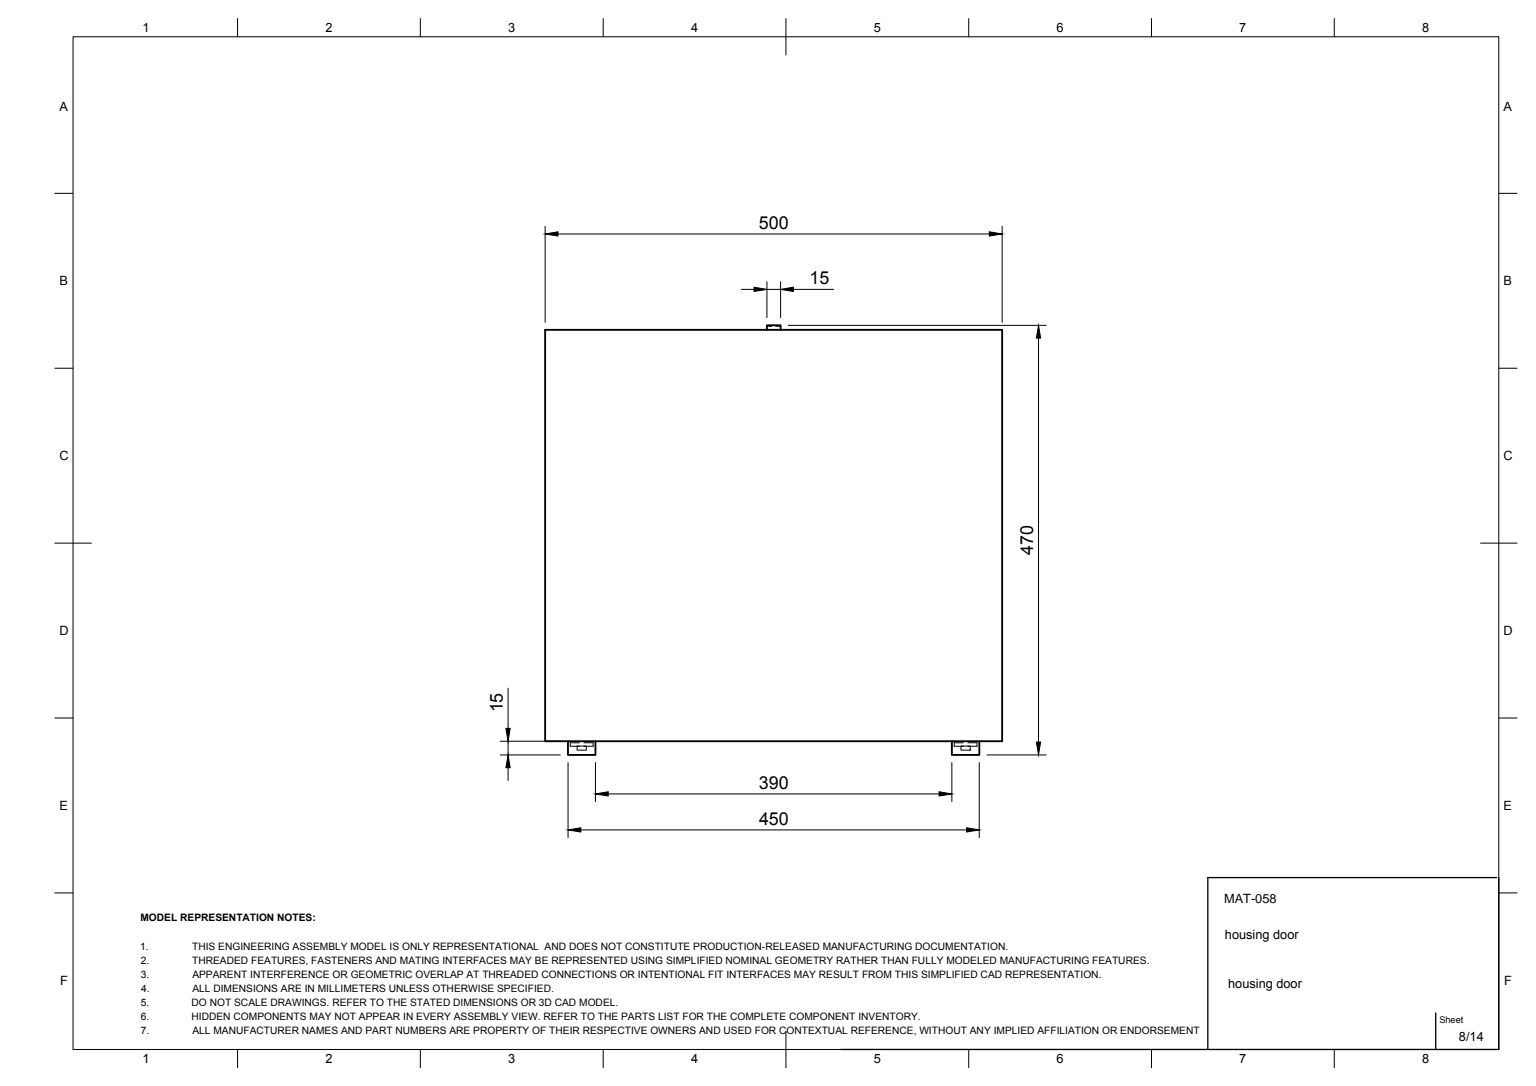
ISO-10303-21;
HEADER;
FILE_DESCRIPTION (('STEP AP214'),
    '1' );
FILE_NAME ('housing door.step',
    '2026-10-21T17:54:40',
    ( '' ),
    ( '' ),
    'SwSTEP 2.0',
    'SolidWorks 2026',
    '' );
FILE_SCHEMA (( 'AUTOMOTIVE_DESIGN' ));
ENDSEC;

DATA;
#107=VECTOR ( 'NONE', #36359, 1000.000000000000000 ) ;
#131=DIRECTION ( 'NONE',  ( -1.000000000000000000, -1.156482317317870492E-16, 0.000000000000000000 ) ) ;
#169=VERTEX_POINT ( 'NONE', #24652 ) ;
#257=LINE ( 'NONE', #31044, #20090 ) ;
#265=LINE ( 'NONE', #19995, #41034 ) ;
#282=DIRECTION ( 'NONE',  ( 0.000000000000000000, -0.000000000000000000, 1.000000000000000000 ) ) ;
#297=VERTEX_POINT ( 'NONE', #25154 ) ;
#306=EDGE_CURVE ( 'NONE', #36749, #10540, #17931, .T. ) ;
#342=ADVANCED_FACE ( 'NONE', ( #29249, #10502, #26150 ), #6152, .F. ) ;
#434=VECTOR ( 'NONE', #13236, 1000.000000000000000 ) ;
#444=FACE_OUTER_BOUND ( 'NONE', #40389, .T. ) ;
#536=EDGE_CURVE ( 'NONE', #38434, #12843, #25274, .T. ) ;
#613=PRODUCT_DEFINITION_CONTEXT ( 'detailed design', #38126, 'design' ) ;
#675=DIRECTION ( 'NONE',  ( 1.000000000000000000, -0.000000000000000000, -0.000000000000000000 ) ) ;
#692=VERTEX_POINT ( 'NONE', #29376 ) ;
#720=LINE ( 'NONE', #35138, #11092 ) ;
#772=DIRECTION ( 'NONE',  ( 0.000000000000000000, 1.000000000000000000, 0.000000000000000000 ) ) ;
#838=DIRECTION ( 'NONE',  ( -1.156482317317870492E-16, 1.000000000000000000, 0.000000000000000000 ) ) ;
#856=ORIENTED_EDGE ( 'NONE', *, *, #7061, .T. ) ;
#953=VERTEX_POINT ( 'NONE', #13403 ) ;
#966=ORIENTED_EDGE ( 'NONE', *, *, #43724, .T. ) ;
#983=VECTOR ( 'NONE', #33572, 1000.000000000000000 ) ;
#1078=( GEOMETRIC_REPRESENTATION_CONTEXT ( 3 ) GLOBAL_UNCERTAINTY_ASSIGNED_CONTEXT ( ( #42989 ) ) GLOBAL_UNIT_ASSIGNED_CONTEXT ( ( #15335, #42505, #10210 ) ) REPRESENTATION_CONTEXT ( 'NONE', 'WORKASPACE' ) );
#1106=FACE_OUTER_BOUND ( 'NONE', #15806, .T. ) ;
#1128=FACE_OUTER_BOUND ( 'NONE', #22979, .T. ) ;
#1143=CARTESIAN_POINT ( 'NONE',  ( 10.00000000000000000, -250.0000000000000000, 225.0000000000000000 ) ) ;
#1154=VECTOR ( 'NONE', #48411, 1000.000000000000000 ) ;
#1155=CARTESIAN_POINT ( 'NONE',  ( 2.499999999999956035, -194.9999999999999716, -224.9999999999999716 ) ) ;
#1205=PLANE ( 'NONE',  #27858 ) ;
#1231=EDGE_CURVE ( 'NONE', #28520, #3732, #42617, .T. ) ;
#1249=DIRECTION ( 'NONE',  ( -0.000000000000000000, -0.000000000000000000, 1.000000000000000000 ) ) ;
#1261=CARTESIAN_POINT ( 'NONE',  ( -8.760073316077686911, -197.4999999999999432, -228.6347188485896140 ) ) ;
#1360=VECTOR ( 'NONE', #42599, 1000.000000000000000 ) ;
#1476=LINE ( 'NONE', #17109, #47212 ) ;
#1506=DIRECTION ( 'NONE',  ( 0.000000000000000000, 0.000000000000000000, 1.000000000000000000 ) ) ;
#1525=ORIENTED_EDGE ( 'NONE', *, *, #2062, .T. ) ;
#1538=LINE ( 'NONE', #40533, #35833 ) ;
#1568=DIRECTION ( 'NONE',  ( 1.000000000000000000, 8.673617379884028076E-17, -0.000000000000000000 ) ) ;
#1577=CARTESIAN_POINT ( 'NONE',  ( 6.204997580903516941, 7.611558401714507482, 225.0000000000000000 ) ) ;
#1621=PLANE ( 'NONE',  #37359 ) ;
#1642=CARTESIAN_POINT ( 'NONE',  ( 2.500000000000000444, 224.9999999999999716, -240.0000000000000000 ) ) ;
#1750=ADVANCED_FACE ( 'NONE', ( #36154 ), #24355, .T. ) ;
#1761=ORIENTED_EDGE ( 'NONE', *, *, #13263, .F. ) ;
#1812=AXIS2_PLACEMENT_3D ( 'NONE', #17777, #25735, #6236 ) ;
#1820=DIRECTION ( 'NONE',  ( 1.000000000000000000, -0.000000000000000000, -0.000000000000000000 ) ) ;
#1892=EDGE_CURVE ( 'NONE', #41332, #44274, #10449, .T. ) ;
#1916=VECTOR ( 'NONE', #48903, 1000.000000000000000 ) ;
#1923=DIRECTION ( 'NONE',  ( 0.000000000000000000, 1.000000000000000000, 0.000000000000000000 ) ) ;
#2017=DIRECTION ( 'NONE',  ( 0.000000000000000000, -1.000000000000000000, 0.000000000000000000 ) ) ;
#2029=DIRECTION ( 'NONE',  ( -1.000000000000000000, 0.000000000000000000, -0.000000000000000000 ) ) ;
#2049=CARTESIAN_POINT ( 'NONE',  ( 7.500000000000000000, 224.9999999999999716, -240.0000000000000000 ) ) ;
#2057=AXIS2_PLACEMENT_3D ( 'NONE', #20662, #32722, #16822 ) ;
#2062=EDGE_CURVE ( 'NONE', #44581, #5075, #47588, .T. ) ;
#2090=FACE_OUTER_BOUND ( 'NONE', #16667, .T. ) ;
#2124=ORIENTED_EDGE ( 'NONE', *, *, #7316, .T. ) ;
#2180=EDGE_CURVE ( 'NONE', #169, #35061, #50319, .T. ) ;
#2216=ORIENTED_EDGE ( 'NONE', *, *, #21301, .F. ) ;
#2233=ORIENTED_EDGE ( 'NONE', *, *, #16780, .F. ) ;
#2234=ADVANCED_FACE ( 'NONE', ( #38594 ), #34751, .T. ) ;
#2362=CARTESIAN_POINT ( 'NONE',  ( -4.999999999999948486, -204.9999999999999716, -234.7500000000000000 ) ) ;
#2397=EDGE_LOOP ( 'NONE', ( #43510, #31402, #50616, #4938 ) ) ;
#2414=VERTEX_POINT ( 'NONE', #19238 ) ;
#2509=LINE ( 'NONE', #25356, #48276 ) ;
#2601=VERTEX_POINT ( 'NONE', #27716 ) ;
#2611=CARTESIAN_POINT ( 'NONE',  ( 4.204997580903516941, -7.388441598285492518, 229.0000000000000000 ) ) ;
#2649=DIRECTION ( 'NONE',  ( 0.000000000000000000, -0.000000000000000000, 1.000000000000000000 ) ) ;
#2666=EDGE_LOOP ( 'NONE', ( #26311, #43649, #8617, #21048 ) ) ;
#2736=PLANE ( 'NONE',  #28390 ) ;
#2783=ORIENTED_EDGE ( 'NONE', *, *, #20337, .F. ) ;
#2843=LINE ( 'NONE', #46433, #10000 ) ;
#2855=VECTOR ( 'NONE', #2017, 1000.000000000000000 ) ;
#2865=VECTOR ( 'NONE', #35878, 1000.000000000000000 ) ;
#2880=VERTEX_POINT ( 'NONE', #11947 ) ;
#3028=CARTESIAN_POINT ( 'NONE',  ( -22.82242230425432439, -2.816136035261162185, 226.0000000000000000 ) ) ;
#3077=ORIENTED_EDGE ( 'NONE', *, *, #19358, .F. ) ;
#3156=VERTEX_POINT ( 'NONE', #34744 ) ;
#3185=LINE ( 'NONE', #27833, #40241 ) ;
#3357=ORIENTED_EDGE ( 'NONE', *, *, #36236, .F. ) ;
#3367=LINE ( 'NONE', #34699, #44682 ) ;
#3415=CARTESIAN_POINT ( 'NONE',  ( -22.82242230425432439, -2.816136035261162185, 229.0000000000000000 ) ) ;
#3446=VERTEX_POINT ( 'NONE', #28795 ) ;
#3504=CARTESIAN_POINT ( 'NONE',  ( 2.500000000000000444, 224.9999999999999716, -240.0000000000000000 ) ) ;
#3509=DIRECTION ( 'NONE',  ( -1.156482317317870492E-16, 1.000000000000000000, 0.000000000000000000 ) ) ;
#3532=EDGE_LOOP ( 'NONE', ( #13431, #22172, #30047, #39452 ) ) ;
#3567=EDGE_CURVE ( 'NONE', #3732, #45897, #46674, .T. ) ;
#3641=AXIS2_PLACEMENT_3D ( 'NONE', #40376, #16766, #8571 ) ;
#3642=CARTESIAN_POINT ( 'NONE',  ( -4.999999999999997335, 204.9999999999999716, -234.7500000000000000 ) ) ;
#3659=ORIENTED_EDGE ( 'NONE', *, *, #49978, .F. ) ;
#3690=CARTESIAN_POINT ( 'NONE',  ( 2.500000000000001776, 214.9999999999999716, -234.7500000000000000 ) ) ;
#3732=VERTEX_POINT ( 'NONE', #47181 ) ;
#3750=LINE ( 'NONE', #31734, #13278 ) ;
#3784=DIRECTION ( 'NONE',  ( -1.000000000000000000, 0.000000000000000000, 0.000000000000000000 ) ) ;
#3839=DIRECTION ( 'NONE',  ( -1.156482317317870492E-16, 1.000000000000000000, 0.000000000000000000 ) ) ;
#3858=DIRECTION ( 'NONE',  ( -0.000000000000000000, 1.000000000000000000, 0.000000000000000000 ) ) ;
#3871=PLANE ( 'NONE',  #11659 ) ;
#3881=PLANE ( 'NONE',  #7841 ) ;
#3891=EDGE_CURVE ( 'NONE', #27411, #18811, #40534, .T. ) ;
#3986=EDGE_CURVE ( 'NONE', #17007, #4976, #15098, .T. ) ;
#4136=CARTESIAN_POINT ( 'NONE',  ( 4.204997580903516941, -7.388441598285492518, 229.0000000000000000 ) ) ;
#4192=EDGE_CURVE ( 'NONE', #26282, #2880, #7924, .T. ) ;
#4231=VECTOR ( 'NONE', #24839, 1000.000000000000000 ) ;
#4341=EDGE_CURVE ( 'NONE', #22510, #5553, #36863, .T. ) ;
#4359=CARTESIAN_POINT ( 'NONE',  ( 4.204997580903515164, -7.388441598285492518, 229.0000000000000000 ) ) ;
#4372=FACE_OUTER_BOUND ( 'NONE', #5239, .T. ) ;
#4545=ORIENTED_EDGE ( 'NONE', *, *, #25529, .T. ) ;
#4570=DIRECTION ( 'NONE',  ( -1.445602896647339410E-16, -1.000000000000000000, -0.000000000000000000 ) ) ;
#4620=ORIENTED_EDGE ( 'NONE', *, *, #5814, .T. ) ;
#4643=FACE_OUTER_BOUND ( 'NONE', #22886, .T. ) ;
#4647=VECTOR ( 'NONE', #1923, 1000.000000000000000 ) ;
#4742=LINE ( 'NONE', #47550, #10008 ) ;
#4752=EDGE_LOOP ( 'NONE', ( #20974, #12743, #21409, #26520 ) ) ;
#4768=LINE ( 'NONE', #15816, #17470 ) ;
#4857=ORIENTED_EDGE ( 'NONE', *, *, #10866, .F. ) ;
#4894=DIRECTION ( 'NONE',  ( 0.000000000000000000, 0.000000000000000000, -1.000000000000000000 ) ) ;
#4938=ORIENTED_EDGE ( 'NONE', *, *, #6764, .F. ) ;
#4976=VERTEX_POINT ( 'NONE', #2049 ) ;
#4998=VECTOR ( 'NONE', #29646, 1000.000000000000000 ) ;
#5035=EDGE_LOOP ( 'NONE', ( #12053, #2783, #27028, #33906 ) ) ;
#5052=VERTEX_POINT ( 'NONE', #42794 ) ;
#5075=VERTEX_POINT ( 'NONE', #31025 ) ;
#5193=DIRECTION ( 'NONE',  ( -1.000000000000000000, 0.000000000000000000, 0.000000000000000000 ) ) ;
#5206=LINE ( 'NONE', #20851, #28066 ) ;
#5239=EDGE_LOOP ( 'NONE', ( #45106, #33408, #44020, #33929 ) ) ;
#5289=APPLICATION_CONTEXT ( 'automotive_design' ) ;
#5291=VERTEX_POINT ( 'NONE', #41228 ) ;
#5307=VERTEX_POINT ( 'NONE', #13016 ) ;
#5329=LINE ( 'NONE', #29437, #38449 ) ;
#5330=LINE ( 'NONE', #20729, #45365 ) ;
#5331=AXIS2_PLACEMENT_3D ( 'NONE', #44627, #1568, #5655 ) ;
#5338=CIRCLE ( 'NONE', #38104, 1.880036658038868103 ) ;
#5379=CARTESIAN_POINT ( 'NONE',  ( -8.760073316077734873, 222.4999999999999716, -228.6347188485896140 ) ) ;
#5407=ORIENTED_EDGE ( 'NONE', *, *, #2180, .F. ) ;
#5435=FACE_OUTER_BOUND ( 'NONE', #31932, .T. ) ;
#5466=CARTESIAN_POINT ( 'NONE',  ( 4.204997580903516941, 7.611558401714507482, 229.0000000000000000 ) ) ;
#5471=CARTESIAN_POINT ( 'NONE',  ( -4.999999999999948486, -204.9999999999999716, -234.7500000000000000 ) ) ;
#5481=EDGE_CURVE ( 'NONE', #10540, #15922, #15557, .T. ) ;
#5492=VECTOR ( 'NONE', #44100, 1000.000000000000000 ) ;
#5506=PLANE ( 'NONE',  #6884 ) ;
#5507=EDGE_CURVE ( 'NONE', #2601, #43558, #3750, .T. ) ;
#5553=VERTEX_POINT ( 'NONE', #20920 ) ;
#5559=EDGE_CURVE ( 'NONE', #15591, #13831, #33489, .T. ) ;
#5616=DIRECTION ( 'NONE',  ( 1.000000000000000000, 0.000000000000000000, -0.000000000000000000 ) ) ;
#5655=DIRECTION ( 'NONE',  ( -8.673617379884028076E-17, 1.000000000000000000, 0.000000000000000000 ) ) ;
#5737=ORIENTED_EDGE ( 'NONE', *, *, #39075, .F. ) ;
#5814=EDGE_CURVE ( 'NONE', #3446, #692, #48217, .T. ) ;
#5862=CARTESIAN_POINT ( 'NONE',  ( 10.00000000000000000, -250.0000000000000000, 225.0000000000000000 ) ) ;
#5922=DIRECTION ( 'NONE',  ( 1.000000000000000000, 0.000000000000000000, 0.000000000000000000 ) ) ;
#5952=DIRECTION ( 'NONE',  ( 1.000000000000000000, 0.000000000000000000, -0.000000000000000000 ) ) ;
#6047=CARTESIAN_POINT ( 'NONE',  ( 7.499999999999944045, -224.9999999999999716, -240.0000000000000000 ) ) ;
#6093=DIRECTION ( 'NONE',  ( -1.000000000000000000, -0.000000000000000000, -0.000000000000000000 ) ) ;
#6112=ORIENTED_EDGE ( 'NONE', *, *, #7061, .F. ) ;
#6152=PLANE ( 'NONE',  #17129 ) ;
#6236=DIRECTION ( 'NONE',  ( 1.000000000000000000, 0.000000000000000000, 0.000000000000000000 ) ) ;
#6260=ORIENTED_EDGE ( 'NONE', *, *, #48354, .T. ) ;
#6264=EDGE_CURVE ( 'NONE', #4976, #14400, #22504, .T. ) ;
#6528=DIRECTION ( 'NONE',  ( 0.000000000000000000, 1.000000000000000000, 0.000000000000000000 ) ) ;
#6543=AXIS2_PLACEMENT_3D ( 'NONE', #40334, #838, #35755 ) ;
#6560=DIRECTION ( 'NONE',  ( 1.000000000000000000, 1.156482317317870492E-16, -0.000000000000000000 ) ) ;
#6576=VECTOR ( 'NONE', #772, 1000.000000000000000 ) ;
#6634=LINE ( 'NONE', #3028, #34072 ) ;
#6647=CARTESIAN_POINT ( 'NONE',  ( 0.000000000000000000, -250.0000000000000000, 225.0000000000000000 ) ) ;
#6649=DIRECTION ( 'NONE',  ( 0.000000000000000000, 0.000000000000000000, 1.000000000000000000 ) ) ;
#6660=AXIS2_PLACEMENT_3D ( 'NONE', #29673, #25323, #45293 ) ;
#6677=EDGE_CURVE ( 'NONE', #29935, #41724, #47839, .T. ) ;
#6764=EDGE_CURVE ( 'NONE', #13831, #12618, #18088, .T. ) ;
#6798=EDGE_CURVE ( 'NONE', #38906, #36749, #3185, .T. ) ;
#6824=EDGE_CURVE ( 'NONE', #47608, #35061, #42694, .T. ) ;
#6867=LINE ( 'NONE', #41011, #31966 ) ;
#6878=ADVANCED_FACE ( 'NONE', ( #30668 ), #15010, .T. ) ;
#6884=AXIS2_PLACEMENT_3D ( 'NONE', #29867, #21403, #32979 ) ;
#6886=DIRECTION ( 'NONE',  ( 0.000000000000000000, 0.000000000000000000, -1.000000000000000000 ) ) ;
#6892=DIRECTION ( 'NONE',  ( -1.000000000000000000, -1.156482317317870492E-16, 0.000000000000000000 ) ) ;
#6971=EDGE_CURVE ( 'NONE', #5052, #12618, #48285, .T. ) ;
#6973=SHAPE_REPRESENTATION_RELATIONSHIP ( 'NONE' , 'NONE' ,  #41838, #12371 ) ;
#6982=ORIENTED_EDGE ( 'NONE', *, *, #1231, .F. ) ;
#7061=EDGE_CURVE ( 'NONE', #16247, #22924, #31945, .T. ) ;
#7147=CARTESIAN_POINT ( 'NONE',  ( -6.880036658038815922, -222.4999999999999716, -228.6347188485896140 ) ) ;
#7156=CARTESIAN_POINT ( 'NONE',  ( 2.499999999999948930, -214.9999999999999716, -230.2499999999999716 ) ) ;
#7175=LINE ( 'NONE', #34141, #29751 ) ;
#7204=ORIENTED_EDGE ( 'NONE', *, *, #50260, .F. ) ;
#7249=CARTESIAN_POINT ( 'NONE',  ( 21.23829395927641883, -7.388441598285492518, 230.0000000000000000 ) ) ;
#7272=CLOSED_SHELL ( 'NONE', ( #18927, #43714, #46822, #342, #22177, #23686, #28004, #1750, #42808, #41362, #48697, #26015, #11744, #28368, #23224, #43415, #21259, #19388, #38381, #50269, #18972, #16515, #14568, #10938, #44795, #41279, #17789, #42653, #44036, #37273, #10881, #10910, #41826, #39115, #8876, #16811, #36818 ) ) ;
#7316=EDGE_CURVE ( 'NONE', #21384, #9147, #38320, .T. ) ;
#7436=CARTESIAN_POINT ( 'NONE',  ( 10.00000000000000000, 249.9999999999999716, -224.9999999999999716 ) ) ;
#7496=DIRECTION ( 'NONE',  ( -1.000000000000000000, 0.000000000000000000, 0.000000000000000000 ) ) ;
#7504=PLANE ( 'NONE',  #45239 ) ;
#7549=ORIENTED_EDGE ( 'NONE', *, *, #2180, .T. ) ;
#7556=ORIENTED_EDGE ( 'NONE', *, *, #13570, .F. ) ;
#7588=VECTOR ( 'NONE', #27240, 1000.000000000000000 ) ;
#7601=EDGE_CURVE ( 'NONE', #17007, #3446, #30468, .T. ) ;
#7614=DIRECTION ( 'NONE',  ( -0.000000000000000000, -1.000000000000000000, -0.000000000000000000 ) ) ;
#7697=EDGE_CURVE ( 'NONE', #44581, #45897, #24309, .T. ) ;
#7779=CARTESIAN_POINT ( 'NONE',  ( 2.499999999999945377, -224.9999999999999716, -240.0000000000000000 ) ) ;
#7813=DIRECTION ( 'NONE',  ( 0.000000000000000000, 0.000000000000000000, 1.000000000000000000 ) ) ;
#7841=AXIS2_PLACEMENT_3D ( 'NONE', #31092, #11332, #39302 ) ;
#7895=DIRECTION ( 'NONE',  ( 1.000000000000000000, -0.000000000000000000, 0.000000000000000000 ) ) ;
#7924=LINE ( 'NONE', #43040, #21221 ) ;
#7957=ORIENTED_EDGE ( 'NONE', *, *, #5507, .T. ) ;
#7958=DIRECTION ( 'NONE',  ( -1.000000000000000000, 0.000000000000000000, 0.000000000000000000 ) ) ;
#8031=LINE ( 'NONE', #7779, #37794 ) ;
#8047=DIRECTION ( 'NONE',  ( 1.156482317317870492E-16, -1.000000000000000000, -0.000000000000000000 ) ) ;
#8219=ORIENTED_EDGE ( 'NONE', *, *, #22109, .F. ) ;
#8269=VECTOR ( 'NONE', #50154, 1000.000000000000000 ) ;
#8273=EDGE_CURVE ( 'NONE', #42084, #26449, #22648, .T. ) ;
#8306=ORIENTED_EDGE ( 'NONE', *, *, #6971, .T. ) ;
#8451=DIRECTION ( 'NONE',  ( -1.156482317317871478E-16, 1.000000000000000000, -0.000000000000000000 ) ) ;
#8503=ORIENTED_EDGE ( 'NONE', *, *, #31244, .T. ) ;
#8538=ORIENTED_EDGE ( 'NONE', *, *, #37613, .F. ) ;
#8571=DIRECTION ( 'NONE',  ( 1.000000000000000000, 0.000000000000000000, -0.000000000000000000 ) ) ;
#8586=EDGE_CURVE ( 'NONE', #26976, #25838, #9043, .T. ) ;
#8613=ORIENTED_EDGE ( 'NONE', *, *, #16112, .F. ) ;
#8615=CARTESIAN_POINT ( 'NONE',  ( -4.999999999999948486, -214.9999999999999716, -230.2499999999999716 ) ) ;
#8617=ORIENTED_EDGE ( 'NONE', *, *, #4192, .T. ) ;
#8681=AXIS2_PLACEMENT_3D ( 'NONE', #28105, #43741, #16556 ) ;
#8685=VECTOR ( 'NONE', #31298, 1000.000000000000000 ) ;
#8714=ORIENTED_EDGE ( 'NONE', *, *, #9844, .T. ) ;
#8715=AXIS2_PLACEMENT_3D ( 'NONE', #21023, #21270, #13060 ) ;
#8773=FACE_BOUND ( 'NONE', #2397, .T. ) ;
#8832=ORIENTED_EDGE ( 'NONE', *, *, #9531, .T. ) ;
#8834=DIRECTION ( 'NONE',  ( -0.000000000000000000, -0.000000000000000000, -1.000000000000000000 ) ) ;
#8845=VECTOR ( 'NONE', #6093, 1000.000000000000000 ) ;
#8876=ADVANCED_FACE ( 'NONE', ( #20512 ), #48421, .F. ) ;
#8899=EDGE_CURVE ( 'NONE', #36068, #2414, #44097, .T. ) ;
#8927=LINE ( 'NONE', #32295, #21492 ) ;
#8946=FACE_OUTER_BOUND ( 'NONE', #24191, .T. ) ;
#8950=ORIENTED_EDGE ( 'NONE', *, *, #32185, .F. ) ;
#8961=ORIENTED_EDGE ( 'NONE', *, *, #7697, .F. ) ;
#9043=CIRCLE ( 'NONE', #6543, 1.880036658038868991 ) ;
#9058=EDGE_LOOP ( 'NONE', ( #13653, #11756, #9966, #7204 ) ) ;
#9069=AXIS2_PLACEMENT_3D ( 'NONE', #47158, #3839, #7958 ) ;
#9147=VERTEX_POINT ( 'NONE', #42027 ) ;
#9158=ORIENTED_EDGE ( 'NONE', *, *, #306, .F. ) ;
#9318=PLANE ( 'NONE',  #11909 ) ;
#9353=CARTESIAN_POINT ( 'NONE',  ( -4.999999999999948486, -204.9999999999999716, -234.7500000000000000 ) ) ;
#9358=ORIENTED_EDGE ( 'NONE', *, *, #6264, .T. ) ;
#9445=( GEOMETRIC_REPRESENTATION_CONTEXT ( 3 ) GLOBAL_UNCERTAINTY_ASSIGNED_CONTEXT ( ( #27008 ) ) GLOBAL_UNIT_ASSIGNED_CONTEXT ( ( #18758, #33681, #45182 ) ) REPRESENTATION_CONTEXT ( 'NONE', 'WORKASPACE' ) );
#9531=EDGE_CURVE ( 'NONE', #26103, #43683, #44893, .T. ) ;
#9576=FACE_OUTER_BOUND ( 'NONE', #11976, .T. ) ;
#9607=ORIENTED_EDGE ( 'NONE', *, *, #45706, .T. ) ;
#9743=AXIS2_PLACEMENT_3D ( 'NONE', #22243, #21987, #37661 ) ;
#9779=DIRECTION ( 'NONE',  ( -1.156482317317870492E-16, 1.000000000000000000, 0.000000000000000000 ) ) ;
#9795=CARTESIAN_POINT ( 'NONE',  ( -4.999999999999948486, -204.9999999999999716, -234.7500000000000000 ) ) ;
#9844=EDGE_CURVE ( 'NONE', #29454, #17433, #49610, .T. ) ;
#9893=EDGE_LOOP ( 'NONE', ( #38931, #16511, #24800, #25278 ) ) ;
#9966=ORIENTED_EDGE ( 'NONE', *, *, #10574, .F. ) ;
#10000=VECTOR ( 'NONE', #50518, 1000.000000000000000 ) ;
#10008=VECTOR ( 'NONE', #16046, 1000.000000000000000 ) ;
#10164=ORIENTED_EDGE ( 'NONE', *, *, #19288, .T. ) ;
#10210=( NAMED_UNIT ( * ) SI_UNIT ( $, .STERADIAN. ) SOLID_ANGLE_UNIT ( ) );
#10235=DIRECTION ( 'NONE',  ( -0.000000000000000000, -0.000000000000000000, 1.000000000000000000 ) ) ;
#10269=ORIENTED_EDGE ( 'NONE', *, *, #50260, .T. ) ;
#10275=LINE ( 'NONE', #48717, #16601 ) ;
#10308=CARTESIAN_POINT ( 'NONE',  ( 7.500000000000000000, 224.9999999999999716, -240.0000000000000000 ) ) ;
#10339=CARTESIAN_POINT ( 'NONE',  ( 7.499999999999944045, -224.9999999999999716, -240.0000000000000000 ) ) ;
#10449=LINE ( 'NONE', #48891, #24716 ) ;
#10485=EDGE_LOOP ( 'NONE', ( #27195, #11760, #38471, #31246 ) ) ;
#10502=FACE_OUTER_BOUND ( 'NONE', #3532, .T. ) ;
#10540=VERTEX_POINT ( 'NONE', #29291 ) ;
#10559=CARTESIAN_POINT ( 'NONE',  ( -4.999999999999948486, -204.9999999999999716, -230.2499999999999716 ) ) ;
#10574=EDGE_CURVE ( 'NONE', #17433, #3732, #43919, .T. ) ;
#10608=ORIENTED_EDGE ( 'NONE', *, *, #33976, .T. ) ;
#10623=PLANE ( 'NONE',  #40550 ) ;
#10677=CARTESIAN_POINT ( 'NONE',  ( -6.880036658038864772, 197.4999999999999432, -228.6347188485896140 ) ) ;
#10807=LINE ( 'NONE', #23115, #32955 ) ;
#10866=EDGE_CURVE ( 'NONE', #15922, #26103, #25136, .T. ) ;
#10871=CARTESIAN_POINT ( 'NONE',  ( 6.204997580903516941, -7.388441598285492518, 230.0000000000000000 ) ) ;
#10881=ADVANCED_FACE ( 'NONE', ( #20764, #13062 ), #28729, .T. ) ;
#10910=ADVANCED_FACE ( 'NONE', ( #24877, #32334 ), #40528, .T. ) ;
#10921=LINE ( 'NONE', #38396, #11054 ) ;
#10938=ADVANCED_FACE ( 'NONE', ( #26124 ), #45605, .F. ) ;
#11054=VECTOR ( 'NONE', #25827, 1000.000000000000000 ) ;
#11071=EDGE_LOOP ( 'NONE', ( #13031, #28160, #2124, #24857, #5737, #16254 ) ) ;
#11092=VECTOR ( 'NONE', #11511, 1000.000000000000000 ) ;
#11217=EDGE_CURVE ( 'NONE', #19049, #22510, #1476, .T. ) ;
#11242=ORIENTED_EDGE ( 'NONE', *, *, #26808, .T. ) ;
#11312=DIRECTION ( 'NONE',  ( 0.000000000000000000, 0.000000000000000000, 1.000000000000000000 ) ) ;
#11332=DIRECTION ( 'NONE',  ( -1.000000000000000000, 0.000000000000000000, 0.000000000000000000 ) ) ;
#11358=ORIENTED_EDGE ( 'NONE', *, *, #39075, .T. ) ;
#11511=DIRECTION ( 'NONE',  ( -1.000000000000000000, -0.000000000000000000, -0.000000000000000000 ) ) ;
#11514=LINE ( 'NONE', #39487, #20879 ) ;
#11659=AXIS2_PLACEMENT_3D ( 'NONE', #4136, #19509, #27234 ) ;
#11664=AXIS2_PLACEMENT_3D ( 'NONE', #20012, #3858, #282 ) ;
#11690=ORIENTED_EDGE ( 'NONE', *, *, #19101, .F. ) ;
#11727=PLANE ( 'NONE',  #34672 ) ;
#11744=ADVANCED_FACE ( 'NONE', ( #5435 ), #21339, .F. ) ;
#11746=ORIENTED_EDGE ( 'NONE', *, *, #7316, .F. ) ;
#11756=ORIENTED_EDGE ( 'NONE', *, *, #3567, .F. ) ;
#11760=ORIENTED_EDGE ( 'NONE', *, *, #7601, .F. ) ;
#11797=AXIS2_PLACEMENT_3D ( 'NONE', #44343, #45092, #44840 ) ;
#11893=CARTESIAN_POINT ( 'NONE',  ( 2.499999999999945377, -224.9999999999999716, -240.0000000000000000 ) ) ;
#11909=AXIS2_PLACEMENT_3D ( 'NONE', #16765, #32424, #48018 ) ;
#11947=CARTESIAN_POINT ( 'NONE',  ( -22.82242230425432439, -2.816136035261162185, 230.0000000000000000 ) ) ;
#11968=DIRECTION ( 'NONE',  ( -1.000000000000000000, 0.000000000000000000, 0.000000000000000000 ) ) ;
#11976=EDGE_LOOP ( 'NONE', ( #8832, #50636, #31082, #21291 ) ) ;
#11980=CARTESIAN_POINT ( 'NONE',  ( -4.999999999999997335, 204.9999999999999716, -230.2499999999999716 ) ) ;
#12053=ORIENTED_EDGE ( 'NONE', *, *, #19288, .F. ) ;
#12117=ORIENTED_EDGE ( 'NONE', *, *, #38802, .F. ) ;
#12139=ORIENTED_EDGE ( 'NONE', *, *, #22804, .T. ) ;
#12230=CARTESIAN_POINT ( 'NONE',  ( -7.822422304254325276, -2.816136035261162185, 226.0000000000000000 ) ) ;
#12339=LINE ( 'NONE', #12851, #30480 ) ;
#12371=ADVANCED_BREP_SHAPE_REPRESENTATION ( '', ( #38799, #38969, #38632, #45486 ), #9445 ) ;
#12389=ORIENTED_EDGE ( 'NONE', *, *, #16780, .T. ) ;
#12390=VECTOR ( 'NONE', #36354, 1000.000000000000000 ) ;
#12409=ORIENTED_EDGE ( 'NONE', *, *, #11217, .F. ) ;
#12420=AXIS2_PLACEMENT_3D ( 'NONE', #10339, #33196, #18259 ) ;
#12439=ORIENTED_EDGE ( 'NONE', *, *, #10574, .T. ) ;
#12443=CYLINDRICAL_SURFACE ( 'NONE', #8681, 1.880036658038868103 ) ;
#12456=PLANE ( 'NONE',  #2057 ) ;
#12487=CARTESIAN_POINT ( 'NONE',  ( 6.204997580903516941, 7.611558401714507482, 230.0000000000000000 ) ) ;
#12498=CARTESIAN_POINT ( 'NONE',  ( 21.23829395927641883, 7.611558401714507482, 229.0000000000000000 ) ) ;
#12546=ORIENTED_EDGE ( 'NONE', *, *, #31423, .T. ) ;
#12567=EDGE_CURVE ( 'NONE', #5307, #38906, #48124, .T. ) ;
#12616=CARTESIAN_POINT ( 'NONE',  ( -8.760073316077734873, 222.4999999999999716, -228.6347188485896140 ) ) ;
#12618=VERTEX_POINT ( 'NONE', #24339 ) ;
#12728=DIRECTION ( 'NONE',  ( -1.000000000000000000, 0.000000000000000000, 0.000000000000000000 ) ) ;
#12743=ORIENTED_EDGE ( 'NONE', *, *, #24046, .F. ) ;
#12781=DIRECTION ( 'NONE',  ( 0.000000000000000000, 0.000000000000000000, 1.000000000000000000 ) ) ;
#12843=VERTEX_POINT ( 'NONE', #8615 ) ;
#12844=SHAPE_DEFINITION_REPRESENTATION ( #18341, #41838 ) ;
#12851=CARTESIAN_POINT ( 'NONE',  ( -4.999999999999997335, 214.9999999999999716, -234.7500000000000000 ) ) ;
#12889=PLANE ( 'NONE',  #15753 ) ;
#12899=ORIENTED_EDGE ( 'NONE', *, *, #5507, .F. ) ;
#12905=CARTESIAN_POINT ( 'NONE',  ( 7.499999999999948486, -194.9999999999999716, -224.9999999999999716 ) ) ;
#12916=DIRECTION ( 'NONE',  ( -1.156482317317871478E-16, 1.000000000000000000, -0.000000000000000000 ) ) ;
#13009=CARTESIAN_POINT ( 'NONE',  ( 7.499999999999944045, -224.9999999999999716, -240.0000000000000000 ) ) ;
#13016=CARTESIAN_POINT ( 'NONE',  ( 7.499999999999948486, -194.9999999999999716, -240.0000000000000000 ) ) ;
#13027=CARTESIAN_POINT ( 'NONE',  ( 0.000000000000000000, 0.000000000000000000, 0.000000000000000000 ) ) ;
#13031=ORIENTED_EDGE ( 'NONE', *, *, #40882, .T. ) ;
#13060=DIRECTION ( 'NONE',  ( 0.000000000000000000, 0.000000000000000000, 1.000000000000000000 ) ) ;
#13062=FACE_OUTER_BOUND ( 'NONE', #49543, .T. ) ;
#13084=VECTOR ( 'NONE', #12916, 1000.000000000000000 ) ;
#13180=EDGE_CURVE ( 'NONE', #28520, #44581, #20998, .T. ) ;
#13236=DIRECTION ( 'NONE',  ( -0.000000000000000000, -0.000000000000000000, 1.000000000000000000 ) ) ;
#13248=LINE ( 'NONE', #40215, #35666 ) ;
#13263=EDGE_CURVE ( 'NONE', #35061, #3446, #31807, .T. ) ;
#13278=VECTOR ( 'NONE', #11968, 1000.000000000000000 ) ;
#13350=CARTESIAN_POINT ( 'NONE',  ( -4.999999999999948486, -204.9999999999999716, -230.2499999999999716 ) ) ;
#13382=FACE_OUTER_BOUND ( 'NONE', #21860, .T. ) ;
#13403=CARTESIAN_POINT ( 'NONE',  ( -25.79500241909648395, 7.611558401714507482, 229.0000000000000000 ) ) ;
#13431=ORIENTED_EDGE ( 'NONE', *, *, #8899, .T. ) ;
#13570=EDGE_CURVE ( 'NONE', #5553, #22510, #19602, .T. ) ;
#13640=DIRECTION ( 'NONE',  ( -1.156482317317871478E-16, -1.000000000000000000, 0.000000000000000000 ) ) ;
#13643=ORIENTED_EDGE ( 'NONE', *, *, #8899, .F. ) ;
#13653=ORIENTED_EDGE ( 'NONE', *, *, #43830, .F. ) ;
#13750=LINE ( 'NONE', #45032, #15575 ) ;
#13831=VERTEX_POINT ( 'NONE', #1577 ) ;
#13848=DIRECTION ( 'NONE',  ( -0.000000000000000000, 1.000000000000000000, -0.000000000000000000 ) ) ;
#13955=DIRECTION ( 'NONE',  ( -1.000000000000000000, 0.000000000000000000, 0.000000000000000000 ) ) ;
#13991=DIRECTION ( 'NONE',  ( -1.000000000000000000, -0.000000000000000000, -0.000000000000000000 ) ) ;
#14005=DIRECTION ( 'NONE',  ( -0.000000000000000000, -0.000000000000000000, 1.000000000000000000 ) ) ;
#14187=ORIENTED_EDGE ( 'NONE', *, *, #6824, .F. ) ;
#14201=FACE_BOUND ( 'NONE', #9058, .T. ) ;
#14204=ORIENTED_EDGE ( 'NONE', *, *, #38083, .T. ) ;
#14237=EDGE_LOOP ( 'NONE', ( #27382, #6260, #24483, #11746 ) ) ;
#14258=ORIENTED_EDGE ( 'NONE', *, *, #50091, .T. ) ;
#14267=DIRECTION ( 'NONE',  ( -1.000000000000000000, 0.000000000000000000, 0.000000000000000000 ) ) ;
#14274=ORIENTED_EDGE ( 'NONE', *, *, #36466, .T. ) ;
#14287=DIRECTION ( 'NONE',  ( -0.000000000000000000, -0.000000000000000000, -1.000000000000000000 ) ) ;
#14289=EDGE_CURVE ( 'NONE', #47880, #9147, #2509, .T. ) ;
#14343=EDGE_CURVE ( 'NONE', #42084, #26282, #6867, .T. ) ;
#14383=DIRECTION ( 'NONE',  ( -1.445602896647339410E-16, -1.000000000000000000, -0.000000000000000000 ) ) ;
#14400=VERTEX_POINT ( 'NONE', #30210 ) ;
#14520=PLANE ( 'NONE',  #18514 ) ;
#14568=ADVANCED_FACE ( 'NONE', ( #444 ), #1205, .F. ) ;
#14668=EDGE_LOOP ( 'NONE', ( #4620, #37003, #20697, #35430 ) ) ;
#14696=DIRECTION ( 'NONE',  ( 1.000000000000000000, 0.000000000000000000, 0.000000000000000000 ) ) ;
#14766=CIRCLE ( 'NONE', #9069, 1.880036658038868103 ) ;
#14779=CARTESIAN_POINT ( 'NONE',  ( 7.500000000000000000, 224.9999999999999716, -240.0000000000000000 ) ) ;
#14790=ORIENTED_EDGE ( 'NONE', *, *, #38529, .T. ) ;
#14794=FACE_OUTER_BOUND ( 'NONE', #2666, .T. ) ;
#14798=CARTESIAN_POINT ( 'NONE',  ( 10.00000000000000000, -250.0000000000000000, -224.9999999999999716 ) ) ;
#14799=CARTESIAN_POINT ( 'NONE',  ( 6.204997580903516941, -7.388441598285492518, 229.0000000000000000 ) ) ;
#14951=STYLED_ITEM('',(#50747),#38799);
#14965=ORIENTED_EDGE ( 'NONE', *, *, #34600, .F. ) ;
#15010=PLANE ( 'NONE',  #45950 ) ;
#15098=LINE ( 'NONE', #42534, #25330 ) ;
#15147=ORIENTED_EDGE ( 'NONE', *, *, #20337, .T. ) ;
#15238=DIRECTION ( 'NONE',  ( -1.000000000000000000, 0.000000000000000000, 0.000000000000000000 ) ) ;
#15335=( LENGTH_UNIT ( ) NAMED_UNIT ( * ) SI_UNIT ( .MILLI., .METRE. ) );
#15557=LINE ( 'NONE', #24280, #30509 ) ;
#15575=VECTOR ( 'NONE', #44786, 1000.000000000000000 ) ;
#15591=VERTEX_POINT ( 'NONE', #12487 ) ;
#15642=EDGE_LOOP ( 'NONE', ( #40302, #33952 ) ) ;
#15706=DIRECTION ( 'NONE',  ( -1.000000000000000000, 0.000000000000000000, 0.000000000000000000 ) ) ;
#15753=AXIS2_PLACEMENT_3D ( 'NONE', #11893, #43187, #15995 ) ;
#15799=EDGE_LOOP ( 'NONE', ( #16885, #16989, #26136, #16240 ) ) ;
#15806=EDGE_LOOP ( 'NONE', ( #20910, #47554, #29756, #26789 ) ) ;
#15816=CARTESIAN_POINT ( 'NONE',  ( 7.499999999999948486, -194.9999999999999716, -240.0000000000000000 ) ) ;
#15908=ORIENTED_EDGE ( 'NONE', *, *, #5481, .F. ) ;
#15922=VERTEX_POINT ( 'NONE', #1155 ) ;
#15995=DIRECTION ( 'NONE',  ( 3.614007241618348278E-16, 1.000000000000000000, 0.000000000000000000 ) ) ;
#16045=ORIENTED_EDGE ( 'NONE', *, *, #46519, .T. ) ;
#16046=DIRECTION ( 'NONE',  ( 1.000000000000000000, 0.000000000000000000, 0.000000000000000000 ) ) ;
#16053=ORIENTED_EDGE ( 'NONE', *, *, #27884, .T. ) ;
#16087=FACE_OUTER_BOUND ( 'NONE', #40191, .T. ) ;
#16100=AXIS2_PLACEMENT_3D ( 'NONE', #24947, #9779, #44658 ) ;
#16111=AXIS2_PLACEMENT_3D ( 'NONE', #43616, #43871, #39542 ) ;
#16112=EDGE_CURVE ( 'NONE', #953, #47880, #29597, .T. ) ;
#16134=CARTESIAN_POINT ( 'NONE',  ( -25.79500241909648395, 0.000000000000000000, 0.000000000000000000 ) ) ;
#16146=DIRECTION ( 'NONE',  ( 8.673617379884028076E-17, -1.000000000000000000, 0.000000000000000000 ) ) ;
#16191=ORIENTED_EDGE ( 'NONE', *, *, #43724, .F. ) ;
#16240=ORIENTED_EDGE ( 'NONE', *, *, #44751, .T. ) ;
#16247=VERTEX_POINT ( 'NONE', #19068 ) ;
#16254=ORIENTED_EDGE ( 'NONE', *, *, #6677, .T. ) ;
#16266=DIRECTION ( 'NONE',  ( 0.000000000000000000, -0.000000000000000000, -1.000000000000000000 ) ) ;
#16331=CARTESIAN_POINT ( 'NONE',  ( -6.880036658038864772, 197.4999999999999432, -228.6347188485896140 ) ) ;
#16436=DIRECTION ( 'NONE',  ( -8.673617379884028076E-17, 1.000000000000000000, -0.000000000000000000 ) ) ;
#16511=ORIENTED_EDGE ( 'NONE', *, *, #31423, .F. ) ;
#16512=DIRECTION ( 'NONE',  ( 1.000000000000000000, 1.156482317317870492E-16, -0.000000000000000000 ) ) ;
#16515=ADVANCED_FACE ( 'NONE', ( #38484 ), #49954, .F. ) ;
#16524=FACE_OUTER_BOUND ( 'NONE', #35918, .T. ) ;
#16556=DIRECTION ( 'NONE',  ( 1.000000000000000000, 0.000000000000000000, 0.000000000000000000 ) ) ;
#16590=CARTESIAN_POINT ( 'NONE',  ( 21.23829395927641883, -7.388441598285492518, 229.0000000000000000 ) ) ;
#16601=VECTOR ( 'NONE', #13848, 1000.000000000000000 ) ;
#16635=MECHANICAL_DESIGN_GEOMETRIC_PRESENTATION_REPRESENTATION('',(#24846),#1078);
#16664=DIRECTION ( 'NONE',  ( -0.000000000000000000, 0.000000000000000000, -1.000000000000000000 ) ) ;
#16667=EDGE_LOOP ( 'NONE', ( #20306, #3659, #48679, #35182 ) ) ;
#16721=ORIENTED_EDGE ( 'NONE', *, *, #43830, .T. ) ;
#16740=CARTESIAN_POINT ( 'NONE',  ( -7.822422304254325276, 2.683863964738837371, 226.0000000000000000 ) ) ;
#16765=CARTESIAN_POINT ( 'NONE',  ( -6.880036658038864772, 197.4999999999999432, -228.6347188485896140 ) ) ;
#16766=DIRECTION ( 'NONE',  ( 0.000000000000000000, -0.000000000000000000, 1.000000000000000000 ) ) ;
#16776=EDGE_CURVE ( 'NONE', #3156, #5291, #48885, .T. ) ;
#16780=EDGE_CURVE ( 'NONE', #38434, #18354, #5329, .T. ) ;
#16781=DIRECTION ( 'NONE',  ( -0.000000000000000000, -1.000000000000000000, -0.000000000000000000 ) ) ;
#16811=ADVANCED_FACE ( 'NONE', ( #14794 ), #30973, .F. ) ;
#16822=DIRECTION ( 'NONE',  ( 8.673617379884028076E-17, -1.000000000000000000, 0.000000000000000000 ) ) ;
#16876=CARTESIAN_POINT ( 'NONE',  ( -4.999999999999997335, 214.9999999999999716, -234.7500000000000000 ) ) ;
#16885=ORIENTED_EDGE ( 'NONE', *, *, #40592, .T. ) ;
#16900=VECTOR ( 'NONE', #6560, 1000.000000000000000 ) ;
#16989=ORIENTED_EDGE ( 'NONE', *, *, #44950, .F. ) ;
#17007=VERTEX_POINT ( 'NONE', #35341 ) ;
#17025=DIRECTION ( 'NONE',  ( -0.000000000000000000, -0.000000000000000000, -1.000000000000000000 ) ) ;
#17099=PRODUCT ( 'housing door', 'housing door', '', ( #28999 ) ) ;
#17109=CARTESIAN_POINT ( 'NONE',  ( -4.999999999999999112, 222.4999999999999716, -228.6347188485896140 ) ) ;
#17129=AXIS2_PLACEMENT_3D ( 'NONE', #41799, #6649, #21542 ) ;
#17205=EDGE_CURVE ( 'NONE', #42094, #30761, #49331, .T. ) ;
#17261=PLANE ( 'NONE',  #28867 ) ;
#17330=CARTESIAN_POINT ( 'NONE',  ( 2.500000000000002665, 204.9999999999999716, -230.2499999999999716 ) ) ;
#17371=EDGE_LOOP ( 'NONE', ( #12439, #6982, #34152, #8714 ) ) ;
#17433=VERTEX_POINT ( 'NONE', #3690 ) ;
#17435=EDGE_LOOP ( 'NONE', ( #16721, #3077, #45773, #42995 ) ) ;
#17462=CARTESIAN_POINT ( 'NONE',  ( 10.00000000000000000, -250.0000000000000000, 225.0000000000000000 ) ) ;
#17470=VECTOR ( 'NONE', #675, 1000.000000000000000 ) ;
#17491=ORIENTED_EDGE ( 'NONE', *, *, #14289, .T. ) ;
#17574=DIRECTION ( 'NONE',  ( 0.000000000000000000, 0.000000000000000000, 1.000000000000000000 ) ) ;
#17609=AXIS2_PLACEMENT_3D ( 'NONE', #18358, #34040, #49622 ) ;
#17698=DIRECTION ( 'NONE',  ( -0.000000000000000000, -0.000000000000000000, 1.000000000000000000 ) ) ;
#17725=VECTOR ( 'NONE', #12781, 1000.000000000000000 ) ;
#17737=CARTESIAN_POINT ( 'NONE',  ( -6.880036658038867436, 222.4999999999999716, -228.6347188485896140 ) ) ;
#17777=CARTESIAN_POINT ( 'NONE',  ( -6.880036658038818587, -197.4999999999999432, -228.6347188485896140 ) ) ;
#17782=EDGE_CURVE ( 'NONE', #43683, #10540, #3367, .T. ) ;
#17789=ADVANCED_FACE ( 'NONE', ( #50276 ), #3881, .F. ) ;
#17931=LINE ( 'NONE', #48941, #26125 ) ;
#17957=ORIENTED_EDGE ( 'NONE', *, *, #49935, .F. ) ;
#18088=LINE ( 'NONE', #21686, #4998 ) ;
#18125=EDGE_CURVE ( 'NONE', #30761, #2414, #22814, .T. ) ;
#18146=ORIENTED_EDGE ( 'NONE', *, *, #37334, .T. ) ;
#18257=DIRECTION ( 'NONE',  ( 8.673617379884028076E-17, -1.000000000000000000, 0.000000000000000000 ) ) ;
#18259=DIRECTION ( 'NONE',  ( -1.445602896647339410E-16, -1.000000000000000000, 0.000000000000000000 ) ) ;
#18341=PRODUCT_DEFINITION_SHAPE ( 'NONE', 'NONE',  #47817 ) ;
#18354=VERTEX_POINT ( 'NONE', #26549 ) ;
#18358=CARTESIAN_POINT ( 'NONE',  ( -4.999999999999997335, 204.9999999999999716, -234.7500000000000000 ) ) ;
#18425=PLANE ( 'NONE',  #21783 ) ;
#18426=EDGE_LOOP ( 'NONE', ( #43406, #2233, #27806, #44434 ) ) ;
#18510=ORIENTED_EDGE ( 'NONE', *, *, #31244, .F. ) ;
#18514=AXIS2_PLACEMENT_3D ( 'NONE', #14779, #26334, #21457 ) ;
#18519=CARTESIAN_POINT ( 'NONE',  ( -4.999999999999948486, -204.9999999999999716, -234.7500000000000000 ) ) ;
#18688=ORIENTED_EDGE ( 'NONE', *, *, #13180, .T. ) ;
#18758=( LENGTH_UNIT ( ) NAMED_UNIT ( * ) SI_UNIT ( .MILLI., .METRE. ) );
#18766=PLANE ( 'NONE',  #42012 ) ;
#18778=EDGE_LOOP ( 'NONE', ( #23293, #43419, #34879, #36645 ) ) ;
#18811=VERTEX_POINT ( 'NONE', #43637 ) ;
#18927=ADVANCED_FACE ( 'NONE', ( #32112, #8773 ), #21308, .F. ) ;
#18972=ADVANCED_FACE ( 'NONE', ( #40811 ), #21058, .F. ) ;
#19014=CARTESIAN_POINT ( 'NONE',  ( -4.999999999999995559, 197.4999999999999432, -228.6347188485896140 ) ) ;
#19018=VERTEX_POINT ( 'NONE', #13350 ) ;
#19038=( GEOMETRIC_REPRESENTATION_CONTEXT ( 3 ) GLOBAL_UNCERTAINTY_ASSIGNED_CONTEXT ( ( #19398 ) ) GLOBAL_UNIT_ASSIGNED_CONTEXT ( ( #22317, #46400, #26419 ) ) REPRESENTATION_CONTEXT ( 'NONE', 'WORKASPACE' ) );
#19049=VERTEX_POINT ( 'NONE', #26680 ) ;
#19068=CARTESIAN_POINT ( 'NONE',  ( 10.00000000000000000, 249.9999999999999716, 225.0000000000000000 ) ) ;
#19101=EDGE_CURVE ( 'NONE', #5291, #18354, #257, .T. ) ;
#19238=CARTESIAN_POINT ( 'NONE',  ( 0.000000000000000000, 249.9999999999999716, -224.9999999999999716 ) ) ;
#19288=EDGE_CURVE ( 'NONE', #33612, #25838, #36159, .T. ) ;
#19358=EDGE_CURVE ( 'NONE', #5075, #297, #48150, .T. ) ;
#19388=ADVANCED_FACE ( 'NONE', ( #8946 ), #32310, .F. ) ;
#19398=UNCERTAINTY_MEASURE_WITH_UNIT (LENGTH_MEASURE( 1.000000000000000082E-05 ), #22317, 'distance_accuracy_value', 'NONE');
#19484=VERTEX_POINT ( 'NONE', #22257 ) ;
#19489=CARTESIAN_POINT ( 'NONE',  ( -4.999999999999997335, 204.9999999999999716, -234.7500000000000000 ) ) ;
#19509=DIRECTION ( 'NONE',  ( 1.000000000000000000, 0.000000000000000000, 0.000000000000000000 ) ) ;
#19602=CIRCLE ( 'NONE', #21248, 1.880036658038868991 ) ;
#19611=CARTESIAN_POINT ( 'NONE',  ( -6.880036658038818587, -197.4999999999999432, -228.6347188485896140 ) ) ;
#19639=DIRECTION ( 'NONE',  ( -0.000000000000000000, -0.000000000000000000, 1.000000000000000000 ) ) ;
#19724=DIRECTION ( 'NONE',  ( 0.000000000000000000, 0.000000000000000000, 1.000000000000000000 ) ) ;
#19886=MECHANICAL_DESIGN_GEOMETRIC_PRESENTATION_REPRESENTATION('',(#14951),#35521);
#19950=VECTOR ( 'NONE', #35177, 1000.000000000000000 ) ;
#19995=CARTESIAN_POINT ( 'NONE',  ( 7.500000000000000000, 224.9999999999999716, -224.9999999999999716 ) ) ;
#20012=CARTESIAN_POINT ( 'NONE',  ( -22.82242230425432439, 2.683863964738837371, 226.0000000000000000 ) ) ;
#20072=ADVANCED_FACE ( 'NONE', ( #44234 ), #12443, .T. ) ;
#20090=VECTOR ( 'NONE', #16146, 1000.000000000000000 ) ;
#20194=ORIENTED_EDGE ( 'NONE', *, *, #23938, .T. ) ;
#20214=DIRECTION ( 'NONE',  ( -0.000000000000000000, -1.000000000000000000, -0.000000000000000000 ) ) ;
#20270=DIRECTION ( 'NONE',  ( 0.000000000000000000, 0.000000000000000000, 1.000000000000000000 ) ) ;
#20306=ORIENTED_EDGE ( 'NONE', *, *, #23938, .F. ) ;
#20327=ORIENTED_EDGE ( 'NONE', *, *, #17782, .F. ) ;
#20337=EDGE_CURVE ( 'NONE', #19484, #33612, #44714, .T. ) ;
#20428=CARTESIAN_POINT ( 'NONE',  ( -25.79500241909648395, -7.388441598285492518, 229.0000000000000000 ) ) ;
#20512=FACE_OUTER_BOUND ( 'NONE', #23617, .T. ) ;
#20519=CARTESIAN_POINT ( 'NONE',  ( 6.204997580903516941, 7.611558401714507482, 230.0000000000000000 ) ) ;
#20662=CARTESIAN_POINT ( 'NONE',  ( -4.999999999999967137, -6.505213034912994064E-16, 0.000000000000000000 ) ) ;
#20697=ORIENTED_EDGE ( 'NONE', *, *, #3986, .F. ) ;
#20729=CARTESIAN_POINT ( 'NONE',  ( 7.499999999999996447, 194.9999999999999716, -240.0000000000000000 ) ) ;
#20742=DIRECTION ( 'NONE',  ( 1.000000000000000000, 1.156482317317870492E-16, 0.000000000000000000 ) ) ;
#20764=FACE_BOUND ( 'NONE', #22978, .T. ) ;
#20851=CARTESIAN_POINT ( 'NONE',  ( -4.999999999999948486, -214.9999999999999716, -230.2499999999999716 ) ) ;
#20879=VECTOR ( 'NONE', #34880, 1000.000000000000000 ) ;
#20910=ORIENTED_EDGE ( 'NONE', *, *, #5481, .T. ) ;
#20920=CARTESIAN_POINT ( 'NONE',  ( -8.760073316077733097, 197.4999999999999432, -228.6347188485896140 ) ) ;
#20935=VECTOR ( 'NONE', #40506, 1000.000000000000000 ) ;
#20974=ORIENTED_EDGE ( 'NONE', *, *, #47148, .T. ) ;
#20998=LINE ( 'NONE', #23845, #32734 ) ;
#21005=CARTESIAN_POINT ( 'NONE',  ( -4.999999999999948486, -204.9999999999999716, -234.7500000000000000 ) ) ;
#21023=CARTESIAN_POINT ( 'NONE',  ( 10.00000000000000000, 0.000000000000000000, 0.000000000000000000 ) ) ;
#21025=CARTESIAN_POINT ( 'NONE',  ( 21.23829395927641883, 7.611558401714507482, 230.0000000000000000 ) ) ;
#21030=DIRECTION ( 'NONE',  ( -0.000000000000000000, -0.000000000000000000, 1.000000000000000000 ) ) ;
#21038=DIRECTION ( 'NONE',  ( 1.156482317317870492E-16, -1.000000000000000000, -0.000000000000000000 ) ) ;
#21048=ORIENTED_EDGE ( 'NONE', *, *, #22804, .F. ) ;
#21058=PLANE ( 'NONE',  #5331 ) ;
#21065=ORIENTED_EDGE ( 'NONE', *, *, #49935, .T. ) ;
#21085=DIRECTION ( 'NONE',  ( -1.000000000000000000, 1.156482317317871478E-16, 0.000000000000000000 ) ) ;
#21105=FACE_OUTER_BOUND ( 'NONE', #23992, .T. ) ;
#21131=CARTESIAN_POINT ( 'NONE',  ( 4.204997580903516941, 7.611558401714507482, 229.0000000000000000 ) ) ;
#21221=VECTOR ( 'NONE', #20214, 1000.000000000000000 ) ;
#21245=DIRECTION ( 'NONE',  ( 1.156482317317870492E-16, -1.000000000000000000, 0.000000000000000000 ) ) ;
#21248=AXIS2_PLACEMENT_3D ( 'NONE', #16331, #31748, #12728 ) ;
#21259=ADVANCED_FACE ( 'NONE', ( #30127 ), #37354, .F. ) ;
#21270=DIRECTION ( 'NONE',  ( -1.000000000000000000, 0.000000000000000000, 0.000000000000000000 ) ) ;
#21291=ORIENTED_EDGE ( 'NONE', *, *, #36236, .T. ) ;
#21301=EDGE_CURVE ( 'NONE', #43558, #42084, #21925, .T. ) ;
#21308=PLANE ( 'NONE',  #50329 ) ;
#21331=VECTOR ( 'NONE', #4570, 1000.000000000000000 ) ;
#21339=PLANE ( 'NONE',  #45036 ) ;
#21355=CARTESIAN_POINT ( 'NONE',  ( 4.204997580903516941, -7.388441598285492518, 225.0000000000000000 ) ) ;
#21367=VECTOR ( 'NONE', #1820, 1000.000000000000000 ) ;
#21379=ORIENTED_EDGE ( 'NONE', *, *, #16776, .F. ) ;
#21384=VERTEX_POINT ( 'NONE', #10871 ) ;
#21403=DIRECTION ( 'NONE',  ( 1.000000000000000000, 1.156482317317871478E-16, 0.000000000000000000 ) ) ;
#21409=ORIENTED_EDGE ( 'NONE', *, *, #46519, .F. ) ;
#21457=DIRECTION ( 'NONE',  ( 0.000000000000000000, 0.000000000000000000, -1.000000000000000000 ) ) ;
#21492=VECTOR ( 'NONE', #47883, 1000.000000000000000 ) ;
#21522=LINE ( 'NONE', #20519, #44414 ) ;
#21542=DIRECTION ( 'NONE',  ( 1.000000000000000000, 0.000000000000000000, -0.000000000000000000 ) ) ;
#21651=PLANE ( 'NONE',  #27577 ) ;
#21686=CARTESIAN_POINT ( 'NONE',  ( 4.204997580903516941, 7.611558401714507482, 225.0000000000000000 ) ) ;
#21740=CARTESIAN_POINT ( 'NONE',  ( 10.00000000000000000, 249.9999999999999716, 225.0000000000000000 ) ) ;
#21770=ORIENTED_EDGE ( 'NONE', *, *, #33138, .T. ) ;
#21777=CARTESIAN_POINT ( 'NONE',  ( -4.999999999999948486, -204.9999999999999716, -230.2499999999999716 ) ) ;
#21783=AXIS2_PLACEMENT_3D ( 'NONE', #7147, #33852, #6892 ) ;
#21860=EDGE_LOOP ( 'NONE', ( #25428, #966 ) ) ;
#21912=ORIENTED_EDGE ( 'NONE', *, *, #40592, .F. ) ;
#21915=DIRECTION ( 'NONE',  ( 0.000000000000000000, 1.000000000000000000, 0.000000000000000000 ) ) ;
#21925=LINE ( 'NONE', #45231, #4647 ) ;
#21938=VERTEX_POINT ( 'NONE', #45866 ) ;
#21987=DIRECTION ( 'NONE',  ( -1.000000000000000000, 0.000000000000000000, 0.000000000000000000 ) ) ;
#21991=FACE_OUTER_BOUND ( 'NONE', #9893, .T. ) ;
#22008=CARTESIAN_POINT ( 'NONE',  ( -7.822422304254325276, 2.683863964738837371, 229.0000000000000000 ) ) ;
#22109=EDGE_CURVE ( 'NONE', #18354, #23977, #44548, .T. ) ;
#22128=PLANE ( 'NONE',  #12420 ) ;
#22172=ORIENTED_EDGE ( 'NONE', *, *, #18125, .F. ) ;
#22177=ADVANCED_FACE ( 'NONE', ( #21991 ), #2736, .F. ) ;
#22185=ORIENTED_EDGE ( 'NONE', *, *, #33138, .F. ) ;
#22189=CARTESIAN_POINT ( 'NONE',  ( 10.00000000000000000, 249.9999999999999716, -224.9999999999999716 ) ) ;
#22243=CARTESIAN_POINT ( 'NONE',  ( -22.82242230425432439, -2.816136035261162185, 226.0000000000000000 ) ) ;
#22257=CARTESIAN_POINT ( 'NONE',  ( -4.999999999999950262, -197.4999999999999432, -228.6347188485896140 ) ) ;
#22317=( LENGTH_UNIT ( ) NAMED_UNIT ( * ) SI_UNIT ( .MILLI., .METRE. ) );
#22374=ADVANCED_FACE ( 'NONE', ( #1128 ), #9318, .F. ) ;
#22504=LINE ( 'NONE', #22760, #8269 ) ;
#22510=VERTEX_POINT ( 'NONE', #19014 ) ;
#22648=LINE ( 'NONE', #44958, #39300 ) ;
#22752=LINE ( 'NONE', #14799, #23182 ) ;
#22760=CARTESIAN_POINT ( 'NONE',  ( 7.500000000000000000, 224.9999999999999716, -240.0000000000000000 ) ) ;
#22787=EDGE_LOOP ( 'NONE', ( #14965, #37467, #1761, #5407 ) ) ;
#22801=ADVANCED_FACE ( 'NONE', ( #41778 ), #18425, .F. ) ;
#22804=EDGE_CURVE ( 'NONE', #43558, #2880, #6634, .T. ) ;
#22814=LINE ( 'NONE', #7436, #8685 ) ;
#22864=VECTOR ( 'NONE', #48681, 1000.000000000000000 ) ;
#22886=EDGE_LOOP ( 'NONE', ( #4545, #50440, #8950, #8306 ) ) ;
#22924=VERTEX_POINT ( 'NONE', #43037 ) ;
#22950=DIRECTION ( 'NONE',  ( -0.000000000000000000, -0.000000000000000000, 1.000000000000000000 ) ) ;
#22978=EDGE_LOOP ( 'NONE', ( #31330, #44029, #2216, #12899 ) ) ;
#22979=EDGE_LOOP ( 'NONE', ( #38214, #7556 ) ) ;
#23115=CARTESIAN_POINT ( 'NONE',  ( 6.204997580903516941, -7.388441598285492518, 225.0000000000000000 ) ) ;
#23168=ORIENTED_EDGE ( 'NONE', *, *, #6764, .T. ) ;
#23182=VECTOR ( 'NONE', #14287, 1000.000000000000000 ) ;
#23210=VECTOR ( 'NONE', #31232, 1000.000000000000000 ) ;
#23219=CARTESIAN_POINT ( 'NONE',  ( -25.79500241909648395, 7.611558401714507482, 230.0000000000000000 ) ) ;
#23224=ADVANCED_FACE ( 'NONE', ( #45290 ), #14520, .F. ) ;
#23240=DIRECTION ( 'NONE',  ( 3.614007241618348278E-16, 1.000000000000000000, 0.000000000000000000 ) ) ;
#23286=LINE ( 'NONE', #12498, #2865 ) ;
#23293=ORIENTED_EDGE ( 'NONE', *, *, #43836, .T. ) ;
#23328=EDGE_CURVE ( 'NONE', #26449, #18811, #34542, .T. ) ;
#23391=VECTOR ( 'NONE', #32057, 1000.000000000000000 ) ;
#23427=CARTESIAN_POINT ( 'NONE',  ( -7.822422304254325276, -2.816136035261162185, 230.0000000000000000 ) ) ;
#23533=EDGE_CURVE ( 'NONE', #4976, #692, #37776, .T. ) ;
#23538=DIRECTION ( 'NONE',  ( 0.000000000000000000, 0.000000000000000000, -1.000000000000000000 ) ) ;
#23560=EDGE_LOOP ( 'NONE', ( #31011, #4857, #15908, #20327 ) ) ;
#23581=LINE ( 'NONE', #43827, #45342 ) ;
#23611=CARTESIAN_POINT ( 'NONE',  ( 2.499999999999945377, -224.9999999999999716, -240.0000000000000000 ) ) ;
#23617=EDGE_LOOP ( 'NONE', ( #7957, #12139, #14274, #8538 ) ) ;
#23686=ADVANCED_FACE ( 'NONE', ( #23879 ), #43120, .F. ) ;
#23776=LINE ( 'NONE', #46567, #23210 ) ;
#23798=ORIENTED_EDGE ( 'NONE', *, *, #6798, .F. ) ;
#23845=CARTESIAN_POINT ( 'NONE',  ( -4.999999999999997335, 204.9999999999999716, -234.7500000000000000 ) ) ;
#23879=FACE_OUTER_BOUND ( 'NONE', #4752, .T. ) ;
#23938=EDGE_CURVE ( 'NONE', #27459, #5553, #48183, .T. ) ;
#23977=VERTEX_POINT ( 'NONE', #7156 ) ;
#23980=CARTESIAN_POINT ( 'NONE',  ( 2.500000000000003997, 194.9999999999999716, -240.0000000000000000 ) ) ;
#23992=EDGE_LOOP ( 'NONE', ( #25087, #17491, #14790, #8503 ) ) ;
#24046=EDGE_CURVE ( 'NONE', #42094, #36068, #720, .T. ) ;
#24108=CARTESIAN_POINT ( 'NONE',  ( -4.999999999999997335, 214.9999999999999716, -234.7500000000000000 ) ) ;
#24191=EDGE_LOOP ( 'NONE', ( #10269, #47960, #42692, #32203 ) ) ;
#24280=CARTESIAN_POINT ( 'NONE',  ( 2.499999999999945377, -224.9999999999999716, -224.9999999999999716 ) ) ;
#24309=LINE ( 'NONE', #27645, #50707 ) ;
#24339=CARTESIAN_POINT ( 'NONE',  ( 4.204997580903516941, 7.611558401714507482, 225.0000000000000000 ) ) ;
#24355=PLANE ( 'NONE',  #24921 ) ;
#24382=CARTESIAN_POINT ( 'NONE',  ( 7.499999999999996447, 194.9999999999999716, -240.0000000000000000 ) ) ;
#24384=CARTESIAN_POINT ( 'NONE',  ( 21.23829395927641883, 7.611558401714507482, 229.0000000000000000 ) ) ;
#24458=CARTESIAN_POINT ( 'NONE',  ( 7.499999999999944045, -224.9999999999999716, -224.9999999999999716 ) ) ;
#24478=PLANE ( 'NONE',  #34590 ) ;
#24483=ORIENTED_EDGE ( 'NONE', *, *, #38529, .F. ) ;
#24652=CARTESIAN_POINT ( 'NONE',  ( 7.499999999999996447, 194.9999999999999716, -224.9999999999999716 ) ) ;
#24716=VECTOR ( 'NONE', #25853, 1000.000000000000000 ) ;
#24800=ORIENTED_EDGE ( 'NONE', *, *, #45749, .F. ) ;
#24827=ORIENTED_EDGE ( 'NONE', *, *, #32185, .T. ) ;
#24839=DIRECTION ( 'NONE',  ( -0.000000000000000000, -0.000000000000000000, -1.000000000000000000 ) ) ;
#24846=STYLED_ITEM('',(#50747),#38969);
#24857=ORIENTED_EDGE ( 'NONE', *, *, #14289, .F. ) ;
#24877=FACE_BOUND ( 'NONE', #36984, .T. ) ;
#24921=AXIS2_PLACEMENT_3D ( 'NONE', #13027, #43317, #40245 ) ;
#24947=CARTESIAN_POINT ( 'NONE',  ( -6.880036658038867436, 222.4999999999999716, -228.6347188485896140 ) ) ;
#25087=ORIENTED_EDGE ( 'NONE', *, *, #16112, .T. ) ;
#25122=ORIENTED_EDGE ( 'NONE', *, *, #39750, .F. ) ;
#25136=LINE ( 'NONE', #48173, #5492 ) ;
#25154=CARTESIAN_POINT ( 'NONE',  ( 2.500000000000001776, 214.9999999999999716, -230.2499999999999716 ) ) ;
#25223=CYLINDRICAL_SURFACE ( 'NONE', #1812, 1.880036658038868103 ) ;
#25274=LINE ( 'NONE', #40431, #28693 ) ;
#25278=ORIENTED_EDGE ( 'NONE', *, *, #18125, .T. ) ;
#25291=CLOSED_SHELL ( 'NONE', ( #2234, #35285, #28707, #22374 ) ) ;
#25301=EDGE_CURVE ( 'NONE', #14400, #169, #5330, .T. ) ;
#25323=DIRECTION ( 'NONE',  ( 0.000000000000000000, 0.000000000000000000, -1.000000000000000000 ) ) ;
#25330=VECTOR ( 'NONE', #30758, 1000.000000000000000 ) ;
#25356=CARTESIAN_POINT ( 'NONE',  ( -25.79500241909648395, -7.388441598285492518, 229.0000000000000000 ) ) ;
#25359=AXIS2_PLACEMENT_3D ( 'NONE', #10677, #42471, #14267 ) ;
#25428=ORIENTED_EDGE ( 'NONE', *, *, #49978, .T. ) ;
#25529=EDGE_CURVE ( 'NONE', #12618, #41724, #38170, .T. ) ;
#25577=FACE_OUTER_BOUND ( 'NONE', #50223, .T. ) ;
#25599=LINE ( 'NONE', #21740, #8845 ) ;
#25621=LINE ( 'NONE', #5862, #1154 ) ;
#25715=ORIENTED_EDGE ( 'NONE', *, *, #3891, .F. ) ;
#25733=ORIENTED_EDGE ( 'NONE', *, *, #12567, .T. ) ;
#25735=DIRECTION ( 'NONE',  ( 1.156482317317870492E-16, -1.000000000000000000, -0.000000000000000000 ) ) ;
#25785=CARTESIAN_POINT ( 'NONE',  ( 10.00000000000000000, -250.0000000000000000, -224.9999999999999716 ) ) ;
#25827=DIRECTION ( 'NONE',  ( -0.000000000000000000, -0.000000000000000000, -1.000000000000000000 ) ) ;
#25838=VERTEX_POINT ( 'NONE', #41939 ) ;
#25853=DIRECTION ( 'NONE',  ( -0.000000000000000000, -1.000000000000000000, -0.000000000000000000 ) ) ;
#25870=CARTESIAN_POINT ( 'NONE',  ( -7.822422304254325276, 7.611558401714507482, 229.0000000000000000 ) ) ;
#25945=VECTOR ( 'NONE', #32136, 1000.000000000000000 ) ;
#25980=AXIS2_PLACEMENT_3D ( 'NONE', #21777, #6886, #2029 ) ;
#26013=CARTESIAN_POINT ( 'NONE',  ( -25.79500241909648395, 7.611558401714507482, 229.0000000000000000 ) ) ;
#26015=ADVANCED_FACE ( 'NONE', ( #48019 ), #28820, .F. ) ;
#26103=VERTEX_POINT ( 'NONE', #12905 ) ;
#26124=FACE_OUTER_BOUND ( 'NONE', #15799, .T. ) ;
#26125=VECTOR ( 'NONE', #17698, 1000.000000000000000 ) ;
#26136=ORIENTED_EDGE ( 'NONE', *, *, #38083, .F. ) ;
#26150=FACE_BOUND ( 'NONE', #22787, .T. ) ;
#26227=CARTESIAN_POINT ( 'NONE',  ( -25.79500241909648395, 7.611558401714507482, 229.0000000000000000 ) ) ;
#26277=ORIENTED_EDGE ( 'NONE', *, *, #39909, .T. ) ;
#26282=VERTEX_POINT ( 'NONE', #38801 ) ;
#26311=ORIENTED_EDGE ( 'NONE', *, *, #21301, .T. ) ;
#26317=VECTOR ( 'NONE', #31139, 1000.000000000000000 ) ;
#26334=DIRECTION ( 'NONE',  ( 0.000000000000000000, -1.000000000000000000, -0.000000000000000000 ) ) ;
#26346=ORIENTED_EDGE ( 'NONE', *, *, #45749, .T. ) ;
#26347=AXIS2_PLACEMENT_3D ( 'NONE', #9795, #45863, #5952 ) ;
#26354=CARTESIAN_POINT ( 'NONE',  ( 10.00000000000000000, 249.9999999999999716, 225.0000000000000000 ) ) ;
#26374=AXIS2_PLACEMENT_3D ( 'NONE', #27792, #40356, #5193 ) ;
#26419=( NAMED_UNIT ( * ) SI_UNIT ( $, .STERADIAN. ) SOLID_ANGLE_UNIT ( ) );
#26449=VERTEX_POINT ( 'NONE', #22008 ) ;
#26469=EDGE_CURVE ( 'NONE', #26449, #2601, #41015, .T. ) ;
#26520=ORIENTED_EDGE ( 'NONE', *, *, #39750, .T. ) ;
#26549=CARTESIAN_POINT ( 'NONE',  ( 2.499999999999948930, -214.9999999999999716, -234.7500000000000000 ) ) ;
#26590=ORIENTED_EDGE ( 'NONE', *, *, #13570, .T. ) ;
#26624=CARTESIAN_POINT ( 'NONE',  ( 2.500000000000003997, 194.9999999999999716, -240.0000000000000000 ) ) ;
#26680=CARTESIAN_POINT ( 'NONE',  ( -4.999999999999999112, 222.4999999999999716, -228.6347188485896140 ) ) ;
#26746=FACE_OUTER_BOUND ( 'NONE', #17371, .T. ) ;
#26789=ORIENTED_EDGE ( 'NONE', *, *, #306, .T. ) ;
#26808=EDGE_CURVE ( 'NONE', #38906, #43683, #49104, .T. ) ;
#26859=EDGE_CURVE ( 'NONE', #18811, #26282, #48349, .T. ) ;
#26974=VECTOR ( 'NONE', #8451, 1000.000000000000000 ) ;
#26976=VERTEX_POINT ( 'NONE', #34022 ) ;
#26983=DIRECTION ( 'NONE',  ( 0.000000000000000000, 1.000000000000000000, 0.000000000000000000 ) ) ;
#27008=UNCERTAINTY_MEASURE_WITH_UNIT (LENGTH_MEASURE( 1.000000000000000082E-05 ), #18758, 'distance_accuracy_value', 'NONE');
#27028=ORIENTED_EDGE ( 'NONE', *, *, #44492, .T. ) ;
#27132=LINE ( 'NONE', #16590, #28940 ) ;
#27195=ORIENTED_EDGE ( 'NONE', *, *, #13263, .T. ) ;
#27220=CARTESIAN_POINT ( 'NONE',  ( 2.500000000000002665, 204.9999999999999716, -234.7500000000000000 ) ) ;
#27227=ORIENTED_EDGE ( 'NONE', *, *, #47148, .F. ) ;
#27234=DIRECTION ( 'NONE',  ( 0.000000000000000000, 0.000000000000000000, -1.000000000000000000 ) ) ;
#27240=DIRECTION ( 'NONE',  ( 1.000000000000000000, 1.156482317317870492E-16, -0.000000000000000000 ) ) ;
#27350=ORIENTED_EDGE ( 'NONE', *, *, #27884, .F. ) ;
#27382=ORIENTED_EDGE ( 'NONE', *, *, #36859, .F. ) ;
#27411=VERTEX_POINT ( 'NONE', #23427 ) ;
#27458=VECTOR ( 'NONE', #13991, 1000.000000000000000 ) ;
#27459=VERTEX_POINT ( 'NONE', #12616 ) ;
#27537=EDGE_LOOP ( 'NONE', ( #7549, #14187, #27350, #34330 ) ) ;
#27577=AXIS2_PLACEMENT_3D ( 'NONE', #29861, #21915, #2649 ) ;
#27607=ORIENTED_EDGE ( 'NONE', *, *, #1892, .F. ) ;
#27645=CARTESIAN_POINT ( 'NONE',  ( -4.999999999999997335, 204.9999999999999716, -230.2499999999999716 ) ) ;
#27696=( LENGTH_UNIT ( ) NAMED_UNIT ( * ) SI_UNIT ( .MILLI., .METRE. ) );
#27716=CARTESIAN_POINT ( 'NONE',  ( -7.822422304254325276, -2.816136035261162185, 229.0000000000000000 ) ) ;
#27745=DIRECTION ( 'NONE',  ( 1.000000000000000000, 1.156482317317870492E-16, -0.000000000000000000 ) ) ;
#27792=CARTESIAN_POINT ( 'NONE',  ( -6.880036658038867436, 222.4999999999999716, -228.6347188485896140 ) ) ;
#27806=ORIENTED_EDGE ( 'NONE', *, *, #37334, .F. ) ;
#27833=CARTESIAN_POINT ( 'NONE',  ( 7.499999999999944045, -224.9999999999999716, -240.0000000000000000 ) ) ;
#27858=AXIS2_PLACEMENT_3D ( 'NONE', #32516, #36109, #48094 ) ;
#27884=EDGE_CURVE ( 'NONE', #14400, #47608, #27964, .T. ) ;
#27963=CARTESIAN_POINT ( 'NONE',  ( -22.82242230425432439, -2.816136035261162185, 226.0000000000000000 ) ) ;
#27964=LINE ( 'NONE', #24382, #34950 ) ;
#27967=VECTOR ( 'NONE', #8834, 1000.000000000000000 ) ;
#28000=VECTOR ( 'NONE', #15706, 1000.000000000000000 ) ;
#28004=ADVANCED_FACE ( 'NONE', ( #40275 ), #40776, .F. ) ;
#28006=DIRECTION ( 'NONE',  ( 0.000000000000000000, 0.000000000000000000, 1.000000000000000000 ) ) ;
#28066=VECTOR ( 'NONE', #16512, 1000.000000000000000 ) ;
#28073=LINE ( 'NONE', #5471, #28615 ) ;
#28105=CARTESIAN_POINT ( 'NONE',  ( -6.880036658038818587, -197.4999999999999432, -228.6347188485896140 ) ) ;
#28160=ORIENTED_EDGE ( 'NONE', *, *, #45591, .F. ) ;
#28216=ORIENTED_EDGE ( 'NONE', *, *, #45706, .F. ) ;
#28225=CARTESIAN_POINT ( 'NONE',  ( 0.000000000000000000, -250.0000000000000000, -224.9999999999999716 ) ) ;
#28368=ADVANCED_FACE ( 'NONE', ( #44475 ), #21651, .F. ) ;
#28371=CARTESIAN_POINT ( 'NONE',  ( 0.000000000000000000, 249.9999999999999716, 225.0000000000000000 ) ) ;
#28390=AXIS2_PLACEMENT_3D ( 'NONE', #26354, #37919, #33555 ) ;
#28512=DIRECTION ( 'NONE',  ( -0.000000000000000000, -0.000000000000000000, -1.000000000000000000 ) ) ;
#28520=VERTEX_POINT ( 'NONE', #32144 ) ;
#28615=VECTOR ( 'NONE', #17025, 1000.000000000000000 ) ;
#28693=VECTOR ( 'NONE', #17574, 1000.000000000000000 ) ;
#28707=ADVANCED_FACE ( 'NONE', ( #13382 ), #48493, .T. ) ;
#28729=PLANE ( 'NONE',  #34190 ) ;
#28734=ORIENTED_EDGE ( 'NONE', *, *, #3891, .T. ) ;
#28792=ORIENTED_EDGE ( 'NONE', *, *, #26859, .F. ) ;
#28795=CARTESIAN_POINT ( 'NONE',  ( 2.500000000000000444, 224.9999999999999716, -224.9999999999999716 ) ) ;
#28812=VECTOR ( 'NONE', #16781, 1000.000000000000000 ) ;
#28820=PLANE ( 'NONE',  #3641 ) ;
#28867=AXIS2_PLACEMENT_3D ( 'NONE', #2362, #48511, #45428 ) ;
#28873=DIRECTION ( 'NONE',  ( -0.000000000000000000, -0.000000000000000000, -1.000000000000000000 ) ) ;
#28940=VECTOR ( 'NONE', #39448, 1000.000000000000000 ) ;
#28981=ORIENTED_EDGE ( 'NONE', *, *, #34475, .T. ) ;
#28999=PRODUCT_CONTEXT ( 'NONE', #5289, 'mechanical' ) ;
#29033=DIRECTION ( 'NONE',  ( -1.000000000000000000, 0.000000000000000000, 0.000000000000000000 ) ) ;
#29079=DIRECTION ( 'NONE',  ( -0.000000000000000000, -1.000000000000000000, -0.000000000000000000 ) ) ;
#29142=EDGE_CURVE ( 'NONE', #2414, #41332, #1538, .T. ) ;
#29249=FACE_BOUND ( 'NONE', #23560, .T. ) ;
#29291=CARTESIAN_POINT ( 'NONE',  ( 2.499999999999945377, -224.9999999999999716, -224.9999999999999716 ) ) ;
#29350=EDGE_LOOP ( 'NONE', ( #45164, #8961, #35503, #49915 ) ) ;
#29376=CARTESIAN_POINT ( 'NONE',  ( 7.500000000000000000, 224.9999999999999716, -224.9999999999999716 ) ) ;
#29437=CARTESIAN_POINT ( 'NONE',  ( -4.999999999999948486, -214.9999999999999716, -234.7500000000000000 ) ) ;
#29454=VERTEX_POINT ( 'NONE', #16876 ) ;
#29474=ORIENTED_EDGE ( 'NONE', *, *, #34600, .T. ) ;
#29480=DIRECTION ( 'NONE',  ( 0.000000000000000000, -1.000000000000000000, 0.000000000000000000 ) ) ;
#29597=LINE ( 'NONE', #26013, #49221 ) ;
#29646=DIRECTION ( 'NONE',  ( -1.000000000000000000, -0.000000000000000000, -0.000000000000000000 ) ) ;
#29673=CARTESIAN_POINT ( 'NONE',  ( 0.000000000000000000, 0.000000000000000000, -240.0000000000000000 ) ) ;
#29751=VECTOR ( 'NONE', #45878, 1000.000000000000000 ) ;
#29756=ORIENTED_EDGE ( 'NONE', *, *, #35248, .F. ) ;
#29794=EDGE_LOOP ( 'NONE', ( #30178, #9158, #23798, #11242 ) ) ;
#29861=CARTESIAN_POINT ( 'NONE',  ( 7.499999999999996447, 194.9999999999999716, -240.0000000000000000 ) ) ;
#29867=CARTESIAN_POINT ( 'NONE',  ( 2.500000000000000444, 224.9999999999999716, -240.0000000000000000 ) ) ;
#29877=DIRECTION ( 'NONE',  ( 0.000000000000000000, -0.000000000000000000, 1.000000000000000000 ) ) ;
#29935=VERTEX_POINT ( 'NONE', #4359 ) ;
#29970=DIRECTION ( 'NONE',  ( -0.000000000000000000, -0.000000000000000000, 1.000000000000000000 ) ) ;
#30047=ORIENTED_EDGE ( 'NONE', *, *, #17205, .F. ) ;
#30127=FACE_OUTER_BOUND ( 'NONE', #17435, .T. ) ;
#30131=EDGE_LOOP ( 'NONE', ( #37402, #10164, #26277, #33781 ) ) ;
#30161=CARTESIAN_POINT ( 'NONE',  ( -4.999999999999997335, 214.9999999999999716, -234.7500000000000000 ) ) ;
#30178=ORIENTED_EDGE ( 'NONE', *, *, #17782, .T. ) ;
#30210=CARTESIAN_POINT ( 'NONE',  ( 7.499999999999996447, 194.9999999999999716, -240.0000000000000000 ) ) ;
#30468=LINE ( 'NONE', #3504, #983 ) ;
#30480=VECTOR ( 'NONE', #28512, 1000.000000000000000 ) ;
#30509=VECTOR ( 'NONE', #23240, 1000.000000000000000 ) ;
#30584=LINE ( 'NONE', #26227, #43267 ) ;
#30643=CARTESIAN_POINT ( 'NONE',  ( -4.999999999999997335, 204.9999999999999716, -230.2499999999999716 ) ) ;
#30668=FACE_OUTER_BOUND ( 'NONE', #46900, .T. ) ;
#30730=CARTESIAN_POINT ( 'NONE',  ( 7.499999999999944045, -224.9999999999999716, -240.0000000000000000 ) ) ;
#30758=DIRECTION ( 'NONE',  ( 1.000000000000000000, -0.000000000000000000, -0.000000000000000000 ) ) ;
#30761=VERTEX_POINT ( 'NONE', #22189 ) ;
#30973=PLANE ( 'NONE',  #9743 ) ;
#31011=ORIENTED_EDGE ( 'NONE', *, *, #9531, .F. ) ;
#31025=CARTESIAN_POINT ( 'NONE',  ( -4.999999999999997335, 214.9999999999999716, -230.2499999999999716 ) ) ;
#31044=CARTESIAN_POINT ( 'NONE',  ( 2.500000000000050182, -204.9999999999999716, -234.7500000000000000 ) ) ;
#31082=ORIENTED_EDGE ( 'NONE', *, *, #12567, .F. ) ;
#31091=CARTESIAN_POINT ( 'NONE',  ( -4.999999999999997335, 204.9999999999999716, -234.7500000000000000 ) ) ;
#31092=CARTESIAN_POINT ( 'NONE',  ( 6.204997580903516941, -7.388441598285492518, 229.0000000000000000 ) ) ;
#31139=DIRECTION ( 'NONE',  ( -1.000000000000000000, 0.000000000000000000, 0.000000000000000000 ) ) ;
#31232=DIRECTION ( 'NONE',  ( -0.000000000000000000, -0.000000000000000000, 1.000000000000000000 ) ) ;
#31241=EDGE_LOOP ( 'NONE', ( #39556, #25122, #6112, #12546 ) ) ;
#31244=EDGE_CURVE ( 'NONE', #36272, #953, #30584, .T. ) ;
#31246=ORIENTED_EDGE ( 'NONE', *, *, #6824, .T. ) ;
#31265=DIRECTION ( 'NONE',  ( -1.000000000000000000, 0.000000000000000000, 0.000000000000000000 ) ) ;
#31290=DIRECTION ( 'NONE',  ( -1.000000000000000000, 0.000000000000000000, 0.000000000000000000 ) ) ;
#31298=DIRECTION ( 'NONE',  ( -1.000000000000000000, -0.000000000000000000, -0.000000000000000000 ) ) ;
#31330=ORIENTED_EDGE ( 'NONE', *, *, #26469, .F. ) ;
#31402=ORIENTED_EDGE ( 'NONE', *, *, #40882, .F. ) ;
#31423=EDGE_CURVE ( 'NONE', #16247, #41332, #25599, .T. ) ;
#31429=DIRECTION ( 'NONE',  ( -8.673617379884028076E-17, 1.000000000000000000, -0.000000000000000000 ) ) ;
#31442=ORIENTED_EDGE ( 'NONE', *, *, #4192, .F. ) ;
#31521=CARTESIAN_POINT ( 'NONE',  ( -6.880036658038867436, 222.4999999999999716, -228.6347188485896140 ) ) ;
#31734=CARTESIAN_POINT ( 'NONE',  ( 21.23829395927641883, -2.816136035261161297, 229.0000000000000000 ) ) ;
#31748=DIRECTION ( 'NONE',  ( -1.156482317317870492E-16, 1.000000000000000000, 0.000000000000000000 ) ) ;
#31807=LINE ( 'NONE', #43580, #26974 ) ;
#31842=ORIENTED_EDGE ( 'NONE', *, *, #37613, .T. ) ;
#31923=CARTESIAN_POINT ( 'NONE',  ( 0.000000000000000000, 0.000000000000000000, 0.000000000000000000 ) ) ;
#31932=EDGE_LOOP ( 'NONE', ( #29474, #44487, #42758, #42512 ) ) ;
#31945=LINE ( 'NONE', #1143, #28812 ) ;
#31966=VECTOR ( 'NONE', #29970, 1000.000000000000000 ) ;
#31999=CARTESIAN_POINT ( 'NONE',  ( 4.204997580903516941, -7.388441598285492518, 229.0000000000000000 ) ) ;
#32057=DIRECTION ( 'NONE',  ( 1.156482317317870492E-16, -1.000000000000000000, -0.000000000000000000 ) ) ;
#32112=FACE_OUTER_BOUND ( 'NONE', #31241, .T. ) ;
#32136=DIRECTION ( 'NONE',  ( 8.673617379884028076E-17, -1.000000000000000000, -0.000000000000000000 ) ) ;
#32144=CARTESIAN_POINT ( 'NONE',  ( -4.999999999999997335, 204.9999999999999716, -234.7500000000000000 ) ) ;
#32185=EDGE_CURVE ( 'NONE', #5052, #29935, #45445, .T. ) ;
#32203=ORIENTED_EDGE ( 'NONE', *, *, #19358, .T. ) ;
#32295=CARTESIAN_POINT ( 'NONE',  ( -4.999999999999950262, -197.4999999999999432, -228.6347188485896140 ) ) ;
#32310=PLANE ( 'NONE',  #50363 ) ;
#32334=FACE_OUTER_BOUND ( 'NONE', #14237, .T. ) ;
#32424=DIRECTION ( 'NONE',  ( -1.156482317317870492E-16, 1.000000000000000000, 0.000000000000000000 ) ) ;
#32430=DIRECTION ( 'NONE',  ( 0.000000000000000000, -1.000000000000000000, 0.000000000000000000 ) ) ;
#32516=CARTESIAN_POINT ( 'NONE',  ( -4.999999999999948486, -214.9999999999999716, -234.7500000000000000 ) ) ;
#32566=CARTESIAN_POINT ( 'NONE',  ( -4.999999999999997335, 214.9999999999999716, -230.2499999999999716 ) ) ;
#32636=CYLINDRICAL_SURFACE ( 'NONE', #40234, 1.880036658038868103 ) ;
#32715=FACE_OUTER_BOUND ( 'NONE', #10485, .T. ) ;
#32722=DIRECTION ( 'NONE',  ( -1.000000000000000000, -8.673617379884028076E-17, 0.000000000000000000 ) ) ;
#32734=VECTOR ( 'NONE', #1506, 1000.000000000000000 ) ;
#32830=CARTESIAN_POINT ( 'NONE',  ( 2.499999999999956035, -194.9999999999999716, -240.0000000000000000 ) ) ;
#32889=AXIS2_PLACEMENT_3D ( 'NONE', #50577, #8047, #46733 ) ;
#32955=VECTOR ( 'NONE', #34433, 1000.000000000000000 ) ;
#32979=DIRECTION ( 'NONE',  ( -1.156482317317871478E-16, 1.000000000000000000, 0.000000000000000000 ) ) ;
#32990=CARTESIAN_POINT ( 'NONE',  ( 7.499999999999944045, -224.9999999999999716, -240.0000000000000000 ) ) ;
#32991=CARTESIAN_POINT ( 'NONE',  ( 6.204997580903516941, 7.611558401714507482, 229.0000000000000000 ) ) ;
#33088=VECTOR ( 'NONE', #29033, 1000.000000000000000 ) ;
#33106=ORIENTED_EDGE ( 'NONE', *, *, #5559, .T. ) ;
#33138=EDGE_CURVE ( 'NONE', #19018, #49333, #28073, .T. ) ;
#33196=DIRECTION ( 'NONE',  ( -1.000000000000000000, 1.445602896647339410E-16, 0.000000000000000000 ) ) ;
#33262=AXIS2_PLACEMENT_3D ( 'NONE', #42920, #49563, #15238 ) ;
#33321=DIRECTION ( 'NONE',  ( 0.000000000000000000, 0.000000000000000000, 1.000000000000000000 ) ) ;
#33408=ORIENTED_EDGE ( 'NONE', *, *, #23328, .T. ) ;
#33489=LINE ( 'NONE', #32991, #44405 ) ;
#33513=CARTESIAN_POINT ( 'NONE',  ( -22.82242230425432439, 2.683863964738837371, 230.0000000000000000 ) ) ;
#33555=DIRECTION ( 'NONE',  ( 0.000000000000000000, -0.000000000000000000, -1.000000000000000000 ) ) ;
#33568=LINE ( 'NONE', #21005, #1916 ) ;
#33572=DIRECTION ( 'NONE',  ( -0.000000000000000000, -0.000000000000000000, 1.000000000000000000 ) ) ;
#33612=VERTEX_POINT ( 'NONE', #46013 ) ;
#33681=( NAMED_UNIT ( * ) PLANE_ANGLE_UNIT ( ) SI_UNIT ( $, .RADIAN. ) );
#33691=CARTESIAN_POINT ( 'NONE',  ( 4.204997580903516941, -7.388441598285492518, 229.0000000000000000 ) ) ;
#33742=DIRECTION ( 'NONE',  ( 0.000000000000000000, 1.000000000000000000, 0.000000000000000000 ) ) ;
#33781=ORIENTED_EDGE ( 'NONE', *, *, #44492, .F. ) ;
#33783=CIRCLE ( 'NONE', #26374, 1.880036658038868103 ) ;
#33852=DIRECTION ( 'NONE',  ( -1.156482317317870492E-16, 1.000000000000000000, 0.000000000000000000 ) ) ;
#33906=ORIENTED_EDGE ( 'NONE', *, *, #8586, .T. ) ;
#33929=ORIENTED_EDGE ( 'NONE', *, *, #14343, .F. ) ;
#33952=ORIENTED_EDGE ( 'NONE', *, *, #39909, .F. ) ;
#33976=EDGE_CURVE ( 'NONE', #47608, #17007, #40140, .T. ) ;
#34022=CARTESIAN_POINT ( 'NONE',  ( -4.999999999999947597, -222.4999999999999716, -228.6347188485896140 ) ) ;
#34038=PRODUCT_DEFINITION_FORMATION_WITH_SPECIFIED_SOURCE ( 'ANY', '', #17099, .NOT_KNOWN. ) ;
#34040=DIRECTION ( 'NONE',  ( -1.156482317317870492E-16, 1.000000000000000000, 0.000000000000000000 ) ) ;
#34072=VECTOR ( 'NONE', #10235, 1000.000000000000000 ) ;
#34141=CARTESIAN_POINT ( 'NONE',  ( -7.822422304254325276, -2.816136035261162185, 226.0000000000000000 ) ) ;
#34152=ORIENTED_EDGE ( 'NONE', *, *, #48551, .F. ) ;
#34190=AXIS2_PLACEMENT_3D ( 'NONE', #24384, #16664, #44349 ) ;
#34314=ORIENTED_EDGE ( 'NONE', *, *, #23328, .F. ) ;
#34330=ORIENTED_EDGE ( 'NONE', *, *, #25301, .T. ) ;
#34341=VECTOR ( 'NONE', #27745, 1000.000000000000000 ) ;
#34433=DIRECTION ( 'NONE',  ( 0.000000000000000000, 1.000000000000000000, 0.000000000000000000 ) ) ;
#34446=DIRECTION ( 'NONE',  ( 0.000000000000000000, -0.000000000000000000, 1.000000000000000000 ) ) ;
#34475=EDGE_CURVE ( 'NONE', #33612, #19484, #14766, .T. ) ;
#34542=LINE ( 'NONE', #16740, #48001 ) ;
#34590=AXIS2_PLACEMENT_3D ( 'NONE', #5466, #32430, #16266 ) ;
#34600=EDGE_CURVE ( 'NONE', #692, #169, #265, .T. ) ;
#34672=AXIS2_PLACEMENT_3D ( 'NONE', #12230, #7895, #23538 ) ;
#34699=CARTESIAN_POINT ( 'NONE',  ( 7.499999999999944045, -224.9999999999999716, -224.9999999999999716 ) ) ;
#34744=CARTESIAN_POINT ( 'NONE',  ( 2.499999999999952927, -204.9999999999999716, -230.2499999999999716 ) ) ;
#34751=CYLINDRICAL_SURFACE ( 'NONE', #32889, 1.880036658038868103 ) ;
#34879=ORIENTED_EDGE ( 'NONE', *, *, #36859, .T. ) ;
#34880=DIRECTION ( 'NONE',  ( 1.000000000000000000, 0.000000000000000000, 0.000000000000000000 ) ) ;
#34899=ORIENTED_EDGE ( 'NONE', *, *, #48551, .T. ) ;
#34950=VECTOR ( 'NONE', #39274, 1000.000000000000000 ) ;
#35026=DIRECTION ( 'NONE',  ( 1.000000000000000000, 0.000000000000000000, 0.000000000000000000 ) ) ;
#35061=VERTEX_POINT ( 'NONE', #42645 ) ;
#35135=ORIENTED_EDGE ( 'NONE', *, *, #43048, .T. ) ;
#35138=CARTESIAN_POINT ( 'NONE',  ( 10.00000000000000000, -250.0000000000000000, -224.9999999999999716 ) ) ;
#35177=DIRECTION ( 'NONE',  ( 8.673617379884028076E-17, -1.000000000000000000, -0.000000000000000000 ) ) ;
#35182=ORIENTED_EDGE ( 'NONE', *, *, #4341, .T. ) ;
#35248=EDGE_CURVE ( 'NONE', #36749, #39770, #8031, .T. ) ;
#35285=ADVANCED_FACE ( 'NONE', ( #2090 ), #32636, .T. ) ;
#35289=LINE ( 'NONE', #50354, #40342 ) ;
#35341=CARTESIAN_POINT ( 'NONE',  ( 2.500000000000000444, 224.9999999999999716, -240.0000000000000000 ) ) ;
#35430=ORIENTED_EDGE ( 'NONE', *, *, #7601, .T. ) ;
#35483=STYLED_ITEM('',(#50747),#38632);
#35503=ORIENTED_EDGE ( 'NONE', *, *, #13180, .F. ) ;
#35521=( GEOMETRIC_REPRESENTATION_CONTEXT ( 3 ) GLOBAL_UNCERTAINTY_ASSIGNED_CONTEXT ( ( #50650 ) ) GLOBAL_UNIT_ASSIGNED_CONTEXT ( ( #27696, #39763, #44826 ) ) REPRESENTATION_CONTEXT ( 'NONE', 'WORKASPACE' ) );
#35666=VECTOR ( 'NONE', #14005, 1000.000000000000000 ) ;
#35755=DIRECTION ( 'NONE',  ( -1.000000000000000000, 0.000000000000000000, 0.000000000000000000 ) ) ;
#35798=ORIENTED_EDGE ( 'NONE', *, *, #17205, .T. ) ;
#35833=VECTOR ( 'NONE', #21030, 1000.000000000000000 ) ;
#35872=CARTESIAN_POINT ( 'NONE',  ( 0.000000000000000000, -250.0000000000000000, -224.9999999999999716 ) ) ;
#35878=DIRECTION ( 'NONE',  ( -1.000000000000000000, 0.000000000000000000, 0.000000000000000000 ) ) ;
#35918=EDGE_LOOP ( 'NONE', ( #23168, #50624, #21065, #18510, #48576, #33106 ) ) ;
#35943=EDGE_LOOP ( 'NONE', ( #13643, #27227, #27607, #39315 ) ) ;
#36068=VERTEX_POINT ( 'NONE', #35872 ) ;
#36109=DIRECTION ( 'NONE',  ( -1.156482317317870492E-16, 1.000000000000000000, 0.000000000000000000 ) ) ;
#36136=ORIENTED_EDGE ( 'NONE', *, *, #3986, .T. ) ;
#36154=FACE_OUTER_BOUND ( 'NONE', #35943, .T. ) ;
#36159=LINE ( 'NONE', #1261, #23391 ) ;
#36236=EDGE_CURVE ( 'NONE', #5307, #26103, #13750, .T. ) ;
#36272=VERTEX_POINT ( 'NONE', #23219 ) ;
#36354=DIRECTION ( 'NONE',  ( -8.673617379884028076E-17, 1.000000000000000000, 0.000000000000000000 ) ) ;
#36359=DIRECTION ( 'NONE',  ( -0.000000000000000000, -0.000000000000000000, -1.000000000000000000 ) ) ;
#36466=EDGE_CURVE ( 'NONE', #2880, #27411, #4742, .T. ) ;
#36490=CARTESIAN_POINT ( 'NONE',  ( 0.000000000000000000, -250.0000000000000000, 225.0000000000000000 ) ) ;
#36645=ORIENTED_EDGE ( 'NONE', *, *, #45591, .T. ) ;
#36707=DIRECTION ( 'NONE',  ( 0.000000000000000000, -1.000000000000000000, 0.000000000000000000 ) ) ;
#36749=VERTEX_POINT ( 'NONE', #23611 ) ;
#36763=EDGE_LOOP ( 'NONE', ( #18146, #39503, #14204, #21770 ) ) ;
#36765=CARTESIAN_POINT ( 'NONE',  ( 2.500000000000002665, 204.9999999999999716, -234.7500000000000000 ) ) ;
#36818=ADVANCED_FACE ( 'NONE', ( #4372 ), #39030, .F. ) ;
#36859=EDGE_CURVE ( 'NONE', #15591, #21384, #21522, .T. ) ;
#36863=CIRCLE ( 'NONE', #25359, 1.880036658038868991 ) ;
#36919=DIRECTION ( 'NONE',  ( 1.000000000000000000, 1.156482317317870492E-16, -0.000000000000000000 ) ) ;
#36944=EDGE_LOOP ( 'NONE', ( #37882, #12117, #22185, #41888 ) ) ;
#36984=EDGE_LOOP ( 'NONE', ( #25715, #50524, #31442, #28792 ) ) ;
#37003=ORIENTED_EDGE ( 'NONE', *, *, #23533, .F. ) ;
#37151=PLANE ( 'NONE',  #6660 ) ;
#37213=AXIS2_PLACEMENT_3D ( 'NONE', #42019, #3509, #3784 ) ;
#37264=CARTESIAN_POINT ( 'NONE',  ( 7.499999999999944045, -224.9999999999999716, -224.9999999999999716 ) ) ;
#37273=ADVANCED_FACE ( 'NONE', ( #42116 ), #18766, .F. ) ;
#37334=EDGE_CURVE ( 'NONE', #49333, #38434, #37799, .T. ) ;
#37354=PLANE ( 'NONE',  #42316 ) ;
#37357=EDGE_LOOP ( 'NONE', ( #35798, #26346, #856, #16045 ) ) ;
#37359=AXIS2_PLACEMENT_3D ( 'NONE', #16134, #31290, #19724 ) ;
#37402=ORIENTED_EDGE ( 'NONE', *, *, #34475, .F. ) ;
#37467=ORIENTED_EDGE ( 'NONE', *, *, #5814, .F. ) ;
#37613=EDGE_CURVE ( 'NONE', #2601, #27411, #7175, .T. ) ;
#37661=DIRECTION ( 'NONE',  ( 0.000000000000000000, 0.000000000000000000, 1.000000000000000000 ) ) ;
#37776=LINE ( 'NONE', #10308, #1360 ) ;
#37794=VECTOR ( 'NONE', #43655, 1000.000000000000000 ) ;
#37799=LINE ( 'NONE', #18519, #48531 ) ;
#37882=ORIENTED_EDGE ( 'NONE', *, *, #16776, .T. ) ;
#37897=PLANE ( 'NONE',  #17609 ) ;
#37919=DIRECTION ( 'NONE',  ( 0.000000000000000000, -1.000000000000000000, 0.000000000000000000 ) ) ;
#38072=VECTOR ( 'NONE', #16436, 1000.000000000000000 ) ;
#38083=EDGE_CURVE ( 'NONE', #12843, #19018, #35289, .T. ) ;
#38104=AXIS2_PLACEMENT_3D ( 'NONE', #31521, #47358, #31265 ) ;
#38126=APPLICATION_CONTEXT ( 'automotive_design' ) ;
#38170=LINE ( 'NONE', #49883, #49454 ) ;
#38214=ORIENTED_EDGE ( 'NONE', *, *, #4341, .F. ) ;
#38320=LINE ( 'NONE', #7249, #28000 ) ;
#38381=ADVANCED_FACE ( 'NONE', ( #26746 ), #7504, .F. ) ;
#38396=CARTESIAN_POINT ( 'NONE',  ( 2.500000000000001776, 214.9999999999999716, -234.7500000000000000 ) ) ;
#38434=VERTEX_POINT ( 'NONE', #40072 ) ;
#38449=VECTOR ( 'NONE', #36919, 1000.000000000000000 ) ;
#38471=ORIENTED_EDGE ( 'NONE', *, *, #33976, .F. ) ;
#38484=FACE_OUTER_BOUND ( 'NONE', #18426, .T. ) ;
#38529=EDGE_CURVE ( 'NONE', #9147, #36272, #10275, .T. ) ;
#38594=FACE_OUTER_BOUND ( 'NONE', #49283, .T. ) ;
#38632=MANIFOLD_SOLID_BREP ( 'Cut-Extrude1', #7272 ) ;
#38799=MANIFOLD_SOLID_BREP ( 'Boss-Extrude5', #25291 ) ;
#38801=CARTESIAN_POINT ( 'NONE',  ( -22.82242230425432439, 2.683863964738837371, 230.0000000000000000 ) ) ;
#38802=EDGE_CURVE ( 'NONE', #49333, #5291, #33568, .T. ) ;
#38906=VERTEX_POINT ( 'NONE', #30730 ) ;
#38931=ORIENTED_EDGE ( 'NONE', *, *, #29142, .T. ) ;
#38969=MANIFOLD_SOLID_BREP ( 'Boss-Extrude6', #46569 ) ;
#39030=PLANE ( 'NONE',  #11664 ) ;
#39031=EDGE_LOOP ( 'NONE', ( #1525, #35135, #34899, #18688 ) ) ;
#39075=EDGE_CURVE ( 'NONE', #29935, #47880, #27132, .T. ) ;
#39104=CARTESIAN_POINT ( 'NONE',  ( 7.499999999999996447, 194.9999999999999716, -224.9999999999999716 ) ) ;
#39115=ADVANCED_FACE ( 'NONE', ( #16087 ), #11727, .F. ) ;
#39220=VECTOR ( 'NONE', #29079, 1000.000000000000000 ) ;
#39274=DIRECTION ( 'NONE',  ( -1.000000000000000000, 0.000000000000000000, 0.000000000000000000 ) ) ;
#39300=VECTOR ( 'NONE', #14696, 1000.000000000000000 ) ;
#39302=DIRECTION ( 'NONE',  ( 0.000000000000000000, 0.000000000000000000, 1.000000000000000000 ) ) ;
#39315=ORIENTED_EDGE ( 'NONE', *, *, #29142, .F. ) ;
#39445=VECTOR ( 'NONE', #22950, 1000.000000000000000 ) ;
#39448=DIRECTION ( 'NONE',  ( -1.000000000000000000, 0.000000000000000000, 0.000000000000000000 ) ) ;
#39452=ORIENTED_EDGE ( 'NONE', *, *, #24046, .T. ) ;
#39487=CARTESIAN_POINT ( 'NONE',  ( 4.204997580903516941, -7.388441598285492518, 225.0000000000000000 ) ) ;
#39503=ORIENTED_EDGE ( 'NONE', *, *, #536, .T. ) ;
#39542=DIRECTION ( 'NONE',  ( 0.000000000000000000, -0.000000000000000000, 1.000000000000000000 ) ) ;
#39556=ORIENTED_EDGE ( 'NONE', *, *, #1892, .T. ) ;
#39750=EDGE_CURVE ( 'NONE', #22924, #44274, #25621, .T. ) ;
#39763=( NAMED_UNIT ( * ) PLANE_ANGLE_UNIT ( ) SI_UNIT ( $, .RADIAN. ) );
#39770=VERTEX_POINT ( 'NONE', #32830 ) ;
#39909=EDGE_CURVE ( 'NONE', #25838, #26976, #44541, .T. ) ;
#40072=CARTESIAN_POINT ( 'NONE',  ( -4.999999999999948486, -214.9999999999999716, -234.7500000000000000 ) ) ;
#40140=LINE ( 'NONE', #1642, #13084 ) ;
#40191=EDGE_LOOP ( 'NONE', ( #42423, #31842, #28734, #34314 ) ) ;
#40215=CARTESIAN_POINT ( 'NONE',  ( 2.499999999999956035, -194.9999999999999716, -240.0000000000000000 ) ) ;
#40234=AXIS2_PLACEMENT_3D ( 'NONE', #17737, #43913, #5922 ) ;
#40241=VECTOR ( 'NONE', #43466, 1000.000000000000000 ) ;
#40245=DIRECTION ( 'NONE',  ( 0.000000000000000000, 0.000000000000000000, 1.000000000000000000 ) ) ;
#40247=DIRECTION ( 'NONE',  ( 0.000000000000000000, 0.000000000000000000, -1.000000000000000000 ) ) ;
#40272=FACE_OUTER_BOUND ( 'NONE', #45093, .T. ) ;
#40275=FACE_OUTER_BOUND ( 'NONE', #37357, .T. ) ;
#40302=ORIENTED_EDGE ( 'NONE', *, *, #8586, .F. ) ;
#40316=DIRECTION ( 'NONE',  ( -1.000000000000000000, 0.000000000000000000, -0.000000000000000000 ) ) ;
#40334=CARTESIAN_POINT ( 'NONE',  ( -6.880036658038815922, -222.4999999999999716, -228.6347188485896140 ) ) ;
#40342=VECTOR ( 'NONE', #31429, 1000.000000000000000 ) ;
#40356=DIRECTION ( 'NONE',  ( -1.156482317317870492E-16, 1.000000000000000000, 0.000000000000000000 ) ) ;
#40376=CARTESIAN_POINT ( 'NONE',  ( 0.000000000000000000, 0.000000000000000000, -240.0000000000000000 ) ) ;
#40389=EDGE_LOOP ( 'NONE', ( #49242, #49658, #40653, #12389 ) ) ;
#40431=CARTESIAN_POINT ( 'NONE',  ( -4.999999999999948486, -214.9999999999999716, -234.7500000000000000 ) ) ;
#40506=DIRECTION ( 'NONE',  ( 1.000000000000000000, 1.156482317317870492E-16, -0.000000000000000000 ) ) ;
#40528=PLANE ( 'NONE',  #48849 ) ;
#40533=CARTESIAN_POINT ( 'NONE',  ( 0.000000000000000000, 249.9999999999999716, 225.0000000000000000 ) ) ;
#40534=LINE ( 'NONE', #41037, #22864 ) ;
#40550=AXIS2_PLACEMENT_3D ( 'NONE', #32990, #33742, #29877 ) ;
#40592=EDGE_CURVE ( 'NONE', #23977, #3156, #41046, .T. ) ;
#40653=ORIENTED_EDGE ( 'NONE', *, *, #536, .F. ) ;
#40676=DIRECTION ( 'NONE',  ( 0.000000000000000000, 0.000000000000000000, -1.000000000000000000 ) ) ;
#40776=PLANE ( 'NONE',  #8715 ) ;
#40811=FACE_OUTER_BOUND ( 'NONE', #39031, .T. ) ;
#40838=CARTESIAN_POINT ( 'NONE',  ( 7.500000000000000000, 224.9999999999999716, -240.0000000000000000 ) ) ;
#40882=EDGE_CURVE ( 'NONE', #41724, #21938, #11514, .T. ) ;
#41011=CARTESIAN_POINT ( 'NONE',  ( -22.82242230425432439, 2.683863964738837371, 226.0000000000000000 ) ) ;
#41015=LINE ( 'NONE', #25870, #2855 ) ;
#41034=VECTOR ( 'NONE', #42574, 1000.000000000000000 ) ;
#41037=CARTESIAN_POINT ( 'NONE',  ( -7.822422304254325276, -2.816136035261162185, 230.0000000000000000 ) ) ;
#41046=LINE ( 'NONE', #44858, #38072 ) ;
#41140=EDGE_LOOP ( 'NONE', ( #25733, #47063, #43872, #9607 ) ) ;
#41163=MECHANICAL_DESIGN_GEOMETRIC_PRESENTATION_REPRESENTATION('',(#35483),#19038);
#41228=CARTESIAN_POINT ( 'NONE',  ( 2.500000000000050182, -204.9999999999999716, -234.7500000000000000 ) ) ;
#41279=ADVANCED_FACE ( 'NONE', ( #48066 ), #12456, .T. ) ;
#41332=VERTEX_POINT ( 'NONE', #28371 ) ;
#41362=ADVANCED_FACE ( 'NONE', ( #41931 ), #10623, .F. ) ;
#41654=DIRECTION ( 'NONE',  ( 0.000000000000000000, -1.000000000000000000, 0.000000000000000000 ) ) ;
#41704=VECTOR ( 'NONE', #14383, 1000.000000000000000 ) ;
#41724=VERTEX_POINT ( 'NONE', #21355 ) ;
#41778=FACE_OUTER_BOUND ( 'NONE', #15642, .T. ) ;
#41799=CARTESIAN_POINT ( 'NONE',  ( 10.00000000000000000, -250.0000000000000000, -224.9999999999999716 ) ) ;
#41826=ADVANCED_FACE ( 'NONE', ( #21105 ), #1621, .T. ) ;
#41838=SHAPE_REPRESENTATION ( 'housing door', ( #45486 ), #9445 ) ;
#41872=DIRECTION ( 'NONE',  ( -0.000000000000000000, -0.000000000000000000, -1.000000000000000000 ) ) ;
#41888=ORIENTED_EDGE ( 'NONE', *, *, #44950, .T. ) ;
#41931=FACE_OUTER_BOUND ( 'NONE', #29794, .T. ) ;
#41939=CARTESIAN_POINT ( 'NONE',  ( -8.760073316077685135, -222.4999999999999716, -228.6347188485896140 ) ) ;
#42012=AXIS2_PLACEMENT_3D ( 'NONE', #2611, #26983, #34446 ) ;
#42019=CARTESIAN_POINT ( 'NONE',  ( -6.880036658038815922, -222.4999999999999716, -228.6347188485896140 ) ) ;
#42027=CARTESIAN_POINT ( 'NONE',  ( -25.79500241909648395, -7.388441598285492518, 230.0000000000000000 ) ) ;
#42084=VERTEX_POINT ( 'NONE', #48888 ) ;
#42094=VERTEX_POINT ( 'NONE', #14798 ) ;
#42116=FACE_OUTER_BOUND ( 'NONE', #11071, .T. ) ;
#42316=AXIS2_PLACEMENT_3D ( 'NONE', #45735, #40676, #13955 ) ;
#42423=ORIENTED_EDGE ( 'NONE', *, *, #26469, .T. ) ;
#42471=DIRECTION ( 'NONE',  ( -1.156482317317870492E-16, 1.000000000000000000, 0.000000000000000000 ) ) ;
#42505=( NAMED_UNIT ( * ) PLANE_ANGLE_UNIT ( ) SI_UNIT ( $, .RADIAN. ) );
#42512=ORIENTED_EDGE ( 'NONE', *, *, #23533, .T. ) ;
#42534=CARTESIAN_POINT ( 'NONE',  ( 7.500000000000000000, 224.9999999999999716, -240.0000000000000000 ) ) ;
#42574=DIRECTION ( 'NONE',  ( -1.156482317317871478E-16, -1.000000000000000000, 0.000000000000000000 ) ) ;
#42599=DIRECTION ( 'NONE',  ( -0.000000000000000000, -0.000000000000000000, 1.000000000000000000 ) ) ;
#42617=LINE ( 'NONE', #31091, #34341 ) ;
#42645=CARTESIAN_POINT ( 'NONE',  ( 2.500000000000003997, 194.9999999999999716, -224.9999999999999716 ) ) ;
#42653=ADVANCED_FACE ( 'NONE', ( #16524 ), #24478, .F. ) ;
#42692=ORIENTED_EDGE ( 'NONE', *, *, #43048, .F. ) ;
#42694=LINE ( 'NONE', #23980, #39445 ) ;
#42758=ORIENTED_EDGE ( 'NONE', *, *, #6264, .F. ) ;
#42794=CARTESIAN_POINT ( 'NONE',  ( 4.204997580903516941, 7.611558401714507482, 229.0000000000000000 ) ) ;
#42808=ADVANCED_FACE ( 'NONE', ( #9576 ), #22128, .F. ) ;
#42845=ADVANCED_FACE ( 'NONE', ( #44697 ), #25223, .T. ) ;
#42920=CARTESIAN_POINT ( 'NONE',  ( -6.880036658038818587, -197.4999999999999432, -228.6347188485896140 ) ) ;
#42989=UNCERTAINTY_MEASURE_WITH_UNIT (LENGTH_MEASURE( 1.000000000000000082E-05 ), #15335, 'distance_accuracy_value', 'NONE');
#42995=ORIENTED_EDGE ( 'NONE', *, *, #7697, .T. ) ;
#43037=CARTESIAN_POINT ( 'NONE',  ( 10.00000000000000000, -250.0000000000000000, 225.0000000000000000 ) ) ;
#43040=CARTESIAN_POINT ( 'NONE',  ( -22.82242230425432439, -2.816136035261162185, 230.0000000000000000 ) ) ;
#43048=EDGE_CURVE ( 'NONE', #5075, #29454, #12339, .T. ) ;
#43120=PLANE ( 'NONE',  #16111 ) ;
#43156=DIRECTION ( 'NONE',  ( 1.000000000000000000, 0.000000000000000000, -0.000000000000000000 ) ) ;
#43187=DIRECTION ( 'NONE',  ( 1.000000000000000000, -3.614007241618348278E-16, 0.000000000000000000 ) ) ;
#43196=FACE_OUTER_BOUND ( 'NONE', #36944, .T. ) ;
#43219=DIRECTION ( 'NONE',  ( -1.156482317317870492E-16, 1.000000000000000000, 0.000000000000000000 ) ) ;
#43267=VECTOR ( 'NONE', #41872, 1000.000000000000000 ) ;
#43276=DIRECTION ( 'NONE',  ( 1.000000000000000000, 1.156482317317870492E-16, -0.000000000000000000 ) ) ;
#43317=DIRECTION ( 'NONE',  ( -1.000000000000000000, 0.000000000000000000, 0.000000000000000000 ) ) ;
#43406=ORIENTED_EDGE ( 'NONE', *, *, #19101, .T. ) ;
#43415=ADVANCED_FACE ( 'NONE', ( #25577 ), #37151, .T. ) ;
#43419=ORIENTED_EDGE ( 'NONE', *, *, #5559, .F. ) ;
#43466=DIRECTION ( 'NONE',  ( -1.000000000000000000, 0.000000000000000000, 0.000000000000000000 ) ) ;
#43510=ORIENTED_EDGE ( 'NONE', *, *, #43836, .F. ) ;
#43558=VERTEX_POINT ( 'NONE', #3415 ) ;
#43580=CARTESIAN_POINT ( 'NONE',  ( 2.500000000000000444, 224.9999999999999716, -224.9999999999999716 ) ) ;
#43601=DIRECTION ( 'NONE',  ( 0.000000000000000000, -0.000000000000000000, -1.000000000000000000 ) ) ;
#43616=CARTESIAN_POINT ( 'NONE',  ( 10.00000000000000000, -250.0000000000000000, 225.0000000000000000 ) ) ;
#43637=CARTESIAN_POINT ( 'NONE',  ( -7.822422304254325276, 2.683863964738837371, 230.0000000000000000 ) ) ;
#43649=ORIENTED_EDGE ( 'NONE', *, *, #14343, .T. ) ;
#43655=DIRECTION ( 'NONE',  ( 3.614007241618348278E-16, 1.000000000000000000, 0.000000000000000000 ) ) ;
#43683=VERTEX_POINT ( 'NONE', #24458 ) ;
#43714=ADVANCED_FACE ( 'NONE', ( #1106, #48000 ), #12889, .F. ) ;
#43724=EDGE_CURVE ( 'NONE', #27459, #19049, #33783, .T. ) ;
#43741=DIRECTION ( 'NONE',  ( 1.156482317317870492E-16, -1.000000000000000000, -0.000000000000000000 ) ) ;
#43827=CARTESIAN_POINT ( 'NONE',  ( 10.00000000000000000, -250.0000000000000000, 225.0000000000000000 ) ) ;
#43830=EDGE_CURVE ( 'NONE', #45897, #297, #2843, .T. ) ;
#43836=EDGE_CURVE ( 'NONE', #21938, #13831, #10807, .T. ) ;
#43871=DIRECTION ( 'NONE',  ( -0.000000000000000000, 1.000000000000000000, 0.000000000000000000 ) ) ;
#43872=ORIENTED_EDGE ( 'NONE', *, *, #35248, .T. ) ;
#43913=DIRECTION ( 'NONE',  ( 1.156482317317870492E-16, -1.000000000000000000, -0.000000000000000000 ) ) ;
#43919=LINE ( 'NONE', #36765, #25945 ) ;
#44020=ORIENTED_EDGE ( 'NONE', *, *, #26859, .T. ) ;
#44029=ORIENTED_EDGE ( 'NONE', *, *, #8273, .F. ) ;
#44036=ADVANCED_FACE ( 'NONE', ( #4643 ), #3871, .F. ) ;
#44039=DIRECTION ( 'NONE',  ( 1.156482317317870492E-16, -1.000000000000000000, -0.000000000000000000 ) ) ;
#44097=LINE ( 'NONE', #28225, #6576 ) ;
#44100=DIRECTION ( 'NONE',  ( 1.000000000000000000, -0.000000000000000000, -0.000000000000000000 ) ) ;
#44234=FACE_OUTER_BOUND ( 'NONE', #30131, .T. ) ;
#44274=VERTEX_POINT ( 'NONE', #6647 ) ;
#44308=CARTESIAN_POINT ( 'NONE',  ( 2.500000000000050182, -204.9999999999999716, -234.7500000000000000 ) ) ;
#44343=CARTESIAN_POINT ( 'NONE',  ( 7.499999999999948486, -194.9999999999999716, -240.0000000000000000 ) ) ;
#44349=DIRECTION ( 'NONE',  ( -1.000000000000000000, 0.000000000000000000, 0.000000000000000000 ) ) ;
#44368=ORIENTED_EDGE ( 'NONE', *, *, #10866, .T. ) ;
#44405=VECTOR ( 'NONE', #28873, 1000.000000000000000 ) ;
#44414=VECTOR ( 'NONE', #29480, 1000.000000000000000 ) ;
#44434=ORIENTED_EDGE ( 'NONE', *, *, #38802, .T. ) ;
#44475=FACE_OUTER_BOUND ( 'NONE', #27537, .T. ) ;
#44487=ORIENTED_EDGE ( 'NONE', *, *, #25301, .F. ) ;
#44492=EDGE_CURVE ( 'NONE', #19484, #26976, #8927, .T. ) ;
#44541=CIRCLE ( 'NONE', #37213, 1.880036658038868991 ) ;
#44548=LINE ( 'NONE', #44814, #17725 ) ;
#44581=VERTEX_POINT ( 'NONE', #30643 ) ;
#44627=CARTESIAN_POINT ( 'NONE',  ( -4.999999999999979572, -6.505213034913003924E-16, 0.000000000000000000 ) ) ;
#44658=DIRECTION ( 'NONE',  ( -1.000000000000000000, -1.156482317317870492E-16, 0.000000000000000000 ) ) ;
#44682=VECTOR ( 'NONE', #7496, 1000.000000000000000 ) ;
#44697=FACE_OUTER_BOUND ( 'NONE', #5035, .T. ) ;
#44714=CIRCLE ( 'NONE', #33262, 1.880036658038868103 ) ;
#44751=EDGE_CURVE ( 'NONE', #12843, #23977, #5206, .T. ) ;
#44786=DIRECTION ( 'NONE',  ( -0.000000000000000000, -0.000000000000000000, 1.000000000000000000 ) ) ;
#44795=ADVANCED_FACE ( 'NONE', ( #43196 ), #17261, .F. ) ;
#44814=CARTESIAN_POINT ( 'NONE',  ( 2.500000000000051070, -214.9999999999999716, -234.7500000000000000 ) ) ;
#44826=( NAMED_UNIT ( * ) SI_UNIT ( $, .STERADIAN. ) SOLID_ANGLE_UNIT ( ) );
#44840=DIRECTION ( 'NONE',  ( 0.000000000000000000, 0.000000000000000000, -1.000000000000000000 ) ) ;
#44858=CARTESIAN_POINT ( 'NONE',  ( 2.500000000000050182, -204.9999999999999716, -230.2499999999999716 ) ) ;
#44893=LINE ( 'NONE', #37264, #41704 ) ;
#44950=EDGE_CURVE ( 'NONE', #19018, #3156, #45681, .T. ) ;
#44958=CARTESIAN_POINT ( 'NONE',  ( 21.23829395927641883, 2.683863964738837371, 229.0000000000000000 ) ) ;
#45032=CARTESIAN_POINT ( 'NONE',  ( 7.499999999999948486, -194.9999999999999716, -240.0000000000000000 ) ) ;
#45036=AXIS2_PLACEMENT_3D ( 'NONE', #40838, #21085, #13640 ) ;
#45092=DIRECTION ( 'NONE',  ( 0.000000000000000000, -1.000000000000000000, -0.000000000000000000 ) ) ;
#45093=EDGE_LOOP ( 'NONE', ( #44368, #3357, #28216, #14258 ) ) ;
#45106=ORIENTED_EDGE ( 'NONE', *, *, #8273, .T. ) ;
#45164=ORIENTED_EDGE ( 'NONE', *, *, #3567, .T. ) ;
#45182=( NAMED_UNIT ( * ) SI_UNIT ( $, .STERADIAN. ) SOLID_ANGLE_UNIT ( ) );
#45231=CARTESIAN_POINT ( 'NONE',  ( -22.82242230425432439, 7.611558401714507482, 229.0000000000000000 ) ) ;
#45239=AXIS2_PLACEMENT_3D ( 'NONE', #3642, #28006, #43156 ) ;
#45290=FACE_OUTER_BOUND ( 'NONE', #14668, .T. ) ;
#45293=DIRECTION ( 'NONE',  ( -1.000000000000000000, 0.000000000000000000, 0.000000000000000000 ) ) ;
#45342=VECTOR ( 'NONE', #40247, 1000.000000000000000 ) ;
#45365=VECTOR ( 'NONE', #1249, 1000.000000000000000 ) ;
#45428=DIRECTION ( 'NONE',  ( 1.000000000000000000, 1.156482317317870492E-16, 0.000000000000000000 ) ) ;
#45445=LINE ( 'NONE', #33691, #39220 ) ;
#45486=AXIS2_PLACEMENT_3D ( 'NONE', #31923, #7813, #35026 ) ;
#45591=EDGE_CURVE ( 'NONE', #21384, #21938, #22752, .T. ) ;
#45605=PLANE ( 'NONE',  #25980 ) ;
#45681=LINE ( 'NONE', #10559, #7588 ) ;
#45706=EDGE_CURVE ( 'NONE', #39770, #5307, #4768, .T. ) ;
#45735=CARTESIAN_POINT ( 'NONE',  ( -4.999999999999997335, 204.9999999999999716, -230.2499999999999716 ) ) ;
#45749=EDGE_CURVE ( 'NONE', #30761, #16247, #23776, .T. ) ;
#45773=ORIENTED_EDGE ( 'NONE', *, *, #2062, .F. ) ;
#45863=DIRECTION ( 'NONE',  ( 0.000000000000000000, 0.000000000000000000, 1.000000000000000000 ) ) ;
#45866=CARTESIAN_POINT ( 'NONE',  ( 6.204997580903516941, -7.388441598285492518, 225.0000000000000000 ) ) ;
#45878=DIRECTION ( 'NONE',  ( -0.000000000000000000, -0.000000000000000000, 1.000000000000000000 ) ) ;
#45897=VERTEX_POINT ( 'NONE', #17330 ) ;
#45950=AXIS2_PLACEMENT_3D ( 'NONE', #19611, #43219, #131 ) ;
#46013=CARTESIAN_POINT ( 'NONE',  ( -8.760073316077686911, -197.4999999999999432, -228.6347188485896140 ) ) ;
#46400=( NAMED_UNIT ( * ) PLANE_ANGLE_UNIT ( ) SI_UNIT ( $, .RADIAN. ) );
#46433=CARTESIAN_POINT ( 'NONE',  ( 2.500000000000002665, 204.9999999999999716, -230.2499999999999716 ) ) ;
#46519=EDGE_CURVE ( 'NONE', #22924, #42094, #23581, .T. ) ;
#46567=CARTESIAN_POINT ( 'NONE',  ( 10.00000000000000000, 249.9999999999999716, 225.0000000000000000 ) ) ;
#46569=CLOSED_SHELL ( 'NONE', ( #20072, #42845, #6878, #22801 ) ) ;
#46674=LINE ( 'NONE', #27220, #47706 ) ;
#46685=AXIS2_PLACEMENT_3D ( 'NONE', #27963, #36707, #43601 ) ;
#46733=DIRECTION ( 'NONE',  ( 1.000000000000000000, 0.000000000000000000, 0.000000000000000000 ) ) ;
#46822=ADVANCED_FACE ( 'NONE', ( #32715, #14201 ), #5506, .F. ) ;
#46900=EDGE_LOOP ( 'NONE', ( #15147, #28981 ) ) ;
#47024=VECTOR ( 'NONE', #48224, 1000.000000000000000 ) ;
#47063=ORIENTED_EDGE ( 'NONE', *, *, #6798, .T. ) ;
#47148=EDGE_CURVE ( 'NONE', #44274, #36068, #48472, .T. ) ;
#47158=CARTESIAN_POINT ( 'NONE',  ( -6.880036658038818587, -197.4999999999999432, -228.6347188485896140 ) ) ;
#47181=CARTESIAN_POINT ( 'NONE',  ( 2.500000000000002665, 204.9999999999999716, -234.7500000000000000 ) ) ;
#47212=VECTOR ( 'NONE', #44039, 1000.000000000000000 ) ;
#47358=DIRECTION ( 'NONE',  ( -1.156482317317870492E-16, 1.000000000000000000, 0.000000000000000000 ) ) ;
#47415=LINE ( 'NONE', #19489, #19950 ) ;
#47550=CARTESIAN_POINT ( 'NONE',  ( -22.82242230425432439, -2.816136035261162185, 230.0000000000000000 ) ) ;
#47554=ORIENTED_EDGE ( 'NONE', *, *, #50091, .F. ) ;
#47588=LINE ( 'NONE', #11980, #12390 ) ;
#47608=VERTEX_POINT ( 'NONE', #26624 ) ;
#47706=VECTOR ( 'NONE', #11312, 1000.000000000000000 ) ;
#47817=PRODUCT_DEFINITION ( 'UNKNOWN', '', #34038, #613 ) ;
#47839=LINE ( 'NONE', #31999, #107 ) ;
#47880=VERTEX_POINT ( 'NONE', #20428 ) ;
#47883=DIRECTION ( 'NONE',  ( 1.156482317317870492E-16, -1.000000000000000000, -0.000000000000000000 ) ) ;
#47960=ORIENTED_EDGE ( 'NONE', *, *, #9844, .F. ) ;
#48000=FACE_BOUND ( 'NONE', #49225, .T. ) ;
#48001=VECTOR ( 'NONE', #19639, 1000.000000000000000 ) ;
#48018=DIRECTION ( 'NONE',  ( -1.000000000000000000, -1.156482317317870492E-16, 0.000000000000000000 ) ) ;
#48019=FACE_OUTER_BOUND ( 'NONE', #41140, .T. ) ;
#48066=FACE_OUTER_BOUND ( 'NONE', #36763, .T. ) ;
#48094=DIRECTION ( 'NONE',  ( -1.000000000000000000, -1.156482317317870492E-16, 0.000000000000000000 ) ) ;
#48124=LINE ( 'NONE', #13009, #21331 ) ;
#48150=LINE ( 'NONE', #32566, #20935 ) ;
#48173=CARTESIAN_POINT ( 'NONE',  ( 7.499999999999948486, -194.9999999999999716, -224.9999999999999716 ) ) ;
#48183=LINE ( 'NONE', #5379, #50378 ) ;
#48202=VECTOR ( 'NONE', #6528, 1000.000000000000000 ) ;
#48217=LINE ( 'NONE', #48466, #21367 ) ;
#48224=DIRECTION ( 'NONE',  ( 0.000000000000000000, 0.000000000000000000, -1.000000000000000000 ) ) ;
#48276=VECTOR ( 'NONE', #33321, 1000.000000000000000 ) ;
#48285=LINE ( 'NONE', #21131, #27967 ) ;
#48349=LINE ( 'NONE', #33513, #27458 ) ;
#48354=EDGE_CURVE ( 'NONE', #15591, #36272, #48973, .T. ) ;
#48411=DIRECTION ( 'NONE',  ( -1.000000000000000000, -0.000000000000000000, -0.000000000000000000 ) ) ;
#48421=PLANE ( 'NONE',  #46685 ) ;
#48466=CARTESIAN_POINT ( 'NONE',  ( 7.500000000000000000, 224.9999999999999716, -224.9999999999999716 ) ) ;
#48472=LINE ( 'NONE', #36490, #47024 ) ;
#48479=CARTESIAN_POINT ( 'NONE',  ( 21.23829395927641883, 7.611558401714507482, 230.0000000000000000 ) ) ;
#48493=PLANE ( 'NONE',  #16100 ) ;
#48511=DIRECTION ( 'NONE',  ( 1.156482317317870492E-16, -1.000000000000000000, 0.000000000000000000 ) ) ;
#48531=VECTOR ( 'NONE', #18257, 1000.000000000000000 ) ;
#48551=EDGE_CURVE ( 'NONE', #29454, #28520, #47415, .T. ) ;
#48576=ORIENTED_EDGE ( 'NONE', *, *, #48354, .F. ) ;
#48679=ORIENTED_EDGE ( 'NONE', *, *, #11217, .T. ) ;
#48681=DIRECTION ( 'NONE',  ( 0.000000000000000000, 1.000000000000000000, 0.000000000000000000 ) ) ;
#48697=ADVANCED_FACE ( 'NONE', ( #40272 ), #48918, .F. ) ;
#48717=CARTESIAN_POINT ( 'NONE',  ( -25.79500241909648395, 7.611558401714507482, 230.0000000000000000 ) ) ;
#48849=AXIS2_PLACEMENT_3D ( 'NONE', #21025, #20270, #5616 ) ;
#48885=LINE ( 'NONE', #44308, #4231 ) ;
#48888=CARTESIAN_POINT ( 'NONE',  ( -22.82242230425432439, 2.683863964738837371, 229.0000000000000000 ) ) ;
#48891=CARTESIAN_POINT ( 'NONE',  ( 0.000000000000000000, -250.0000000000000000, 225.0000000000000000 ) ) ;
#48903=DIRECTION ( 'NONE',  ( 1.000000000000000000, 1.156482317317870492E-16, -0.000000000000000000 ) ) ;
#48918=PLANE ( 'NONE',  #11797 ) ;
#48941=CARTESIAN_POINT ( 'NONE',  ( 2.499999999999945377, -224.9999999999999716, -240.0000000000000000 ) ) ;
#48973=LINE ( 'NONE', #48479, #33088 ) ;
#49104=LINE ( 'NONE', #6047, #434 ) ;
#49221=VECTOR ( 'NONE', #41654, 1000.000000000000000 ) ;
#49225=EDGE_LOOP ( 'NONE', ( #11690, #21379, #21912, #8219 ) ) ;
#49242=ORIENTED_EDGE ( 'NONE', *, *, #22109, .T. ) ;
#49283=EDGE_LOOP ( 'NONE', ( #16191, #20194, #26590, #12409 ) ) ;
#49331=LINE ( 'NONE', #25785, #48202 ) ;
#49333=VERTEX_POINT ( 'NONE', #9353 ) ;
#49375=FACE_OUTER_BOUND ( 'NONE', #29350, .T. ) ;
#49454=VECTOR ( 'NONE', #7614, 1000.000000000000000 ) ;
#49543=EDGE_LOOP ( 'NONE', ( #17957, #24827, #11358, #8613 ) ) ;
#49563=DIRECTION ( 'NONE',  ( -1.156482317317870492E-16, 1.000000000000000000, 0.000000000000000000 ) ) ;
#49610=LINE ( 'NONE', #30161, #16900 ) ;
#49622=DIRECTION ( 'NONE',  ( -1.000000000000000000, -1.156482317317870492E-16, 0.000000000000000000 ) ) ;
#49658=ORIENTED_EDGE ( 'NONE', *, *, #44751, .F. ) ;
#49883=CARTESIAN_POINT ( 'NONE',  ( 4.204997580903516941, -7.388441598285492518, 225.0000000000000000 ) ) ;
#49915=ORIENTED_EDGE ( 'NONE', *, *, #1231, .T. ) ;
#49935=EDGE_CURVE ( 'NONE', #5052, #953, #23286, .T. ) ;
#49954=PLANE ( 'NONE',  #26347 ) ;
#49978=EDGE_CURVE ( 'NONE', #19049, #27459, #5338, .T. ) ;
#50091=EDGE_CURVE ( 'NONE', #39770, #15922, #13248, .T. ) ;
#50154=DIRECTION ( 'NONE',  ( -1.156482317317871478E-16, -1.000000000000000000, 0.000000000000000000 ) ) ;
#50223=EDGE_LOOP ( 'NONE', ( #9358, #16053, #10608, #36136 ) ) ;
#50260=EDGE_CURVE ( 'NONE', #297, #17433, #10921, .T. ) ;
#50269=ADVANCED_FACE ( 'NONE', ( #49375 ), #37897, .F. ) ;
#50276=FACE_OUTER_BOUND ( 'NONE', #18778, .T. ) ;
#50319=LINE ( 'NONE', #39104, #26317 ) ;
#50329=AXIS2_PLACEMENT_3D ( 'NONE', #17462, #4894, #40316 ) ;
#50354=CARTESIAN_POINT ( 'NONE',  ( -4.999999999999948486, -204.9999999999999716, -230.2499999999999716 ) ) ;
#50363=AXIS2_PLACEMENT_3D ( 'NONE', #24108, #21245, #20742 ) ;
#50378=VECTOR ( 'NONE', #21038, 1000.000000000000000 ) ;
#50440=ORIENTED_EDGE ( 'NONE', *, *, #6677, .F. ) ;
#50518=DIRECTION ( 'NONE',  ( -8.673617379884028076E-17, 1.000000000000000000, 0.000000000000000000 ) ) ;
#50524=ORIENTED_EDGE ( 'NONE', *, *, #36466, .F. ) ;
#50577=CARTESIAN_POINT ( 'NONE',  ( -6.880036658038867436, 222.4999999999999716, -228.6347188485896140 ) ) ;
#50616=ORIENTED_EDGE ( 'NONE', *, *, #25529, .F. ) ;
#50624=ORIENTED_EDGE ( 'NONE', *, *, #6971, .F. ) ;
#50636=ORIENTED_EDGE ( 'NONE', *, *, #26808, .F. ) ;
#50650=UNCERTAINTY_MEASURE_WITH_UNIT (LENGTH_MEASURE( 1.000000000000000082E-05 ), #27696, 'distance_accuracy_value', 'NONE');
#50707=VECTOR ( 'NONE', #43276, 1000.000000000000000 ) ;
#50741=COLOUR_RGB('Dark Blue',0.08,0.2,0.34);
#50742=FILL_AREA_STYLE_COLOUR('',#50741);
#50743=FILL_AREA_STYLE('',(#50742));
#50744=SURFACE_STYLE_FILL_AREA(#50743);
#50745=SURFACE_SIDE_STYLE('',(#50744));
#50746=SURFACE_STYLE_USAGE(.BOTH.,#50745);
#50747=PRESENTATION_STYLE_ASSIGNMENT((#50746));
ENDSEC;
END-ISO-10303-21;
